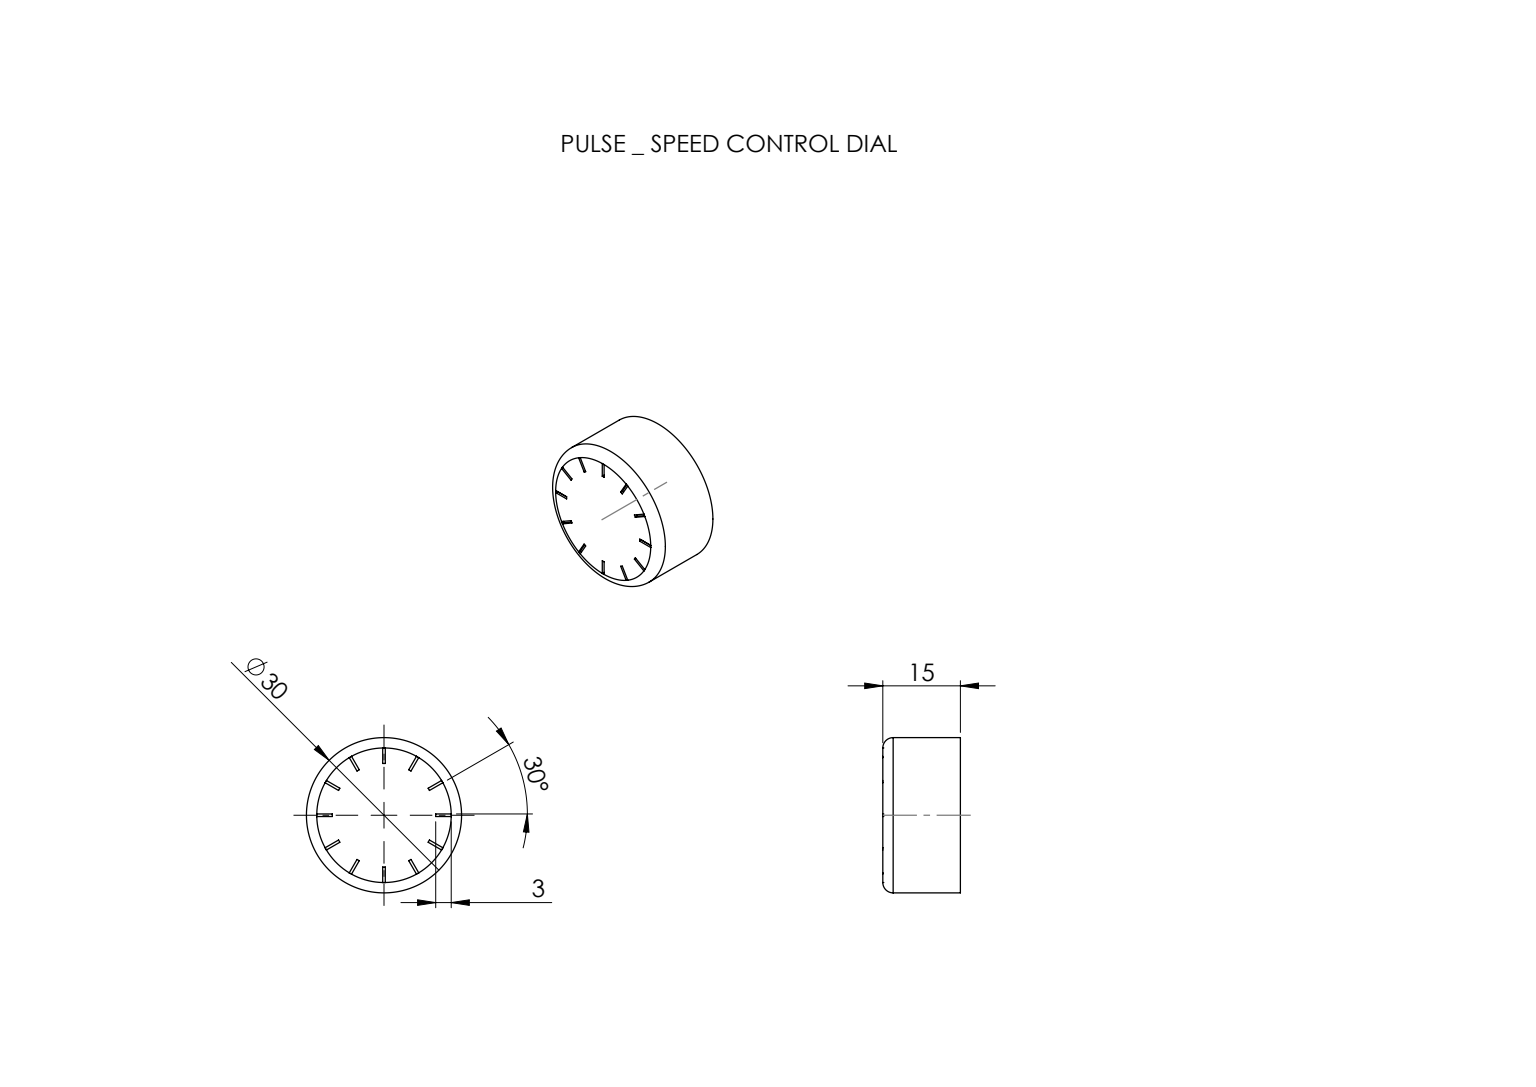
ISO-10303-21;
HEADER;
FILE_DESCRIPTION (('STEP AP214'),
    '1' );
FILE_NAME ('Pulse _ Speed Control Dial.step',
    '2026-10-08T14:59:03',
    ( '' ),
    ( '' ),
    'SwSTEP 2.0',
    'SolidWorks 2026',
    '' );
FILE_SCHEMA (( 'AUTOMOTIVE_DESIGN' ));
ENDSEC;

DATA;
#1=ORIENTED_EDGE ( 'NONE', *, *, #9406, .F. ) ;
#2=CARTESIAN_POINT ( 'NONE',  ( 11.80921887069467324, 30.25000000000018474, 79.50000000000000000 ) ) ;
#6=PLANE ( 'NONE',  #104 ) ;
#11=LINE ( 'NONE', #6448, #10967 ) ;
#15=ORIENTED_EDGE ( 'NONE', *, *, #10225, .T. ) ;
#17=ORIENTED_EDGE ( 'NONE', *, *, #3705, .T. ) ;
#19=EDGE_CURVE ( 'NONE', #6749, #65, #10302, .T. ) ;
#20=DIRECTION ( 'NONE',  ( 0.4999999999999933387, -0.8660254037844424824, 0.000000000000000000 ) ) ;
#21=ORIENTED_EDGE ( 'NONE', *, *, #5442, .F. ) ;
#22=VECTOR ( 'NONE', #10909, 1000.000000000000000 ) ;
#23=CARTESIAN_POINT ( 'NONE',  ( -7.907287480251413925, 18.86666975080236597, 80.00000000000000000 ) ) ;
#27=EDGE_CURVE ( 'NONE', #1251, #10198, #9485, .T. ) ;
#28=ORIENTED_EDGE ( 'NONE', *, *, #12033, .F. ) ;
#37=ORIENTED_EDGE ( 'NONE', *, *, #7691, .T. ) ;
#39=EDGE_CURVE ( 'NONE', #10896, #4898, #9360, .T. ) ;
#40=CARTESIAN_POINT ( 'NONE',  ( -1.440781129305471087, 43.00000000000008527, 80.00000000000000000 ) ) ;
#41=VECTOR ( 'NONE', #11324, 1000.000000000000000 ) ;
#45=VECTOR ( 'NONE', #2118, 1000.000000000000000 ) ;
#46=LINE ( 'NONE', #5798, #12120 ) ;
#47=LINE ( 'NONE', #9767, #6437 ) ;
#65=VERTEX_POINT ( 'NONE', #3417 ) ;
#67=ORIENTED_EDGE ( 'NONE', *, *, #12135, .T. ) ;
#73=CARTESIAN_POINT ( 'NONE',  ( 5.525725221640833240, 18.86666975080242992, 79.50000000000000000 ) ) ;
#78=AXIS2_PLACEMENT_3D ( 'NONE', #1523, #2574, #3573 ) ;
#82=CYLINDRICAL_SURFACE ( 'NONE', #2511, 15.00000000000000000 ) ;
#96=CARTESIAN_POINT ( 'NONE',  ( -1.440781129305282571, 17.00000000000009592, 80.00000000000000000 ) ) ;
#100=ORIENTED_EDGE ( 'NONE', *, *, #2094, .T. ) ;
#104=AXIS2_PLACEMENT_3D ( 'NONE', #11679, #5881, #9664 ) ;
#105=ORIENTED_EDGE ( 'NONE', *, *, #968, .F. ) ;
#110=DIRECTION ( 'NONE',  ( -0.8660254037844363761, 0.5000000000000038858, 0.000000000000000000 ) ) ;
#118=COLOUR_RGB ( '', 0.09019608, 0.27058824, 0.51372549) ;
#135=PLANE ( 'NONE',  #4004 ) ;
#139=ORIENTED_EDGE ( 'NONE', *, *, #323, .F. ) ;
#150=CARTESIAN_POINT ( 'NONE',  ( -0.9407811293052614765, 20.00000000000009237, 79.50000000000000000 ) ) ;
#156=ORIENTED_EDGE ( 'NONE', *, *, #11948, .T. ) ;
#159=CARTESIAN_POINT ( 'NONE',  ( 9.942549119892305498, 36.71650635094628967, 79.50000000000000000 ) ) ;
#160=MECHANICAL_DESIGN_GEOMETRIC_PRESENTATION_REPRESENTATION('',(#10913),#2162);
#162=ORIENTED_EDGE ( 'NONE', *, *, #3844, .F. ) ;
#168=ORIENTED_EDGE ( 'NONE', *, *, #9268, .F. ) ;
#169=CARTESIAN_POINT ( 'NONE',  ( -9.976035167149731819, 34.78349364905394481, 80.00000000000000000 ) ) ;
#171=LINE ( 'NONE', #7782, #5342 ) ;
#175=EDGE_CURVE ( 'NONE', #10718, #2926, #1576, .T. ) ;
#180=CARTESIAN_POINT ( 'NONE',  ( 11.80921887069467324, 30.00000000000008882, 80.00000000000000000 ) ) ;
#186=ORIENTED_EDGE ( 'NONE', *, *, #175, .F. ) ;
#187=DIRECTION ( 'NONE',  ( -1.000000000000000000, 0.000000000000000000, -0.000000000000000000 ) ) ;
#191=DIRECTION ( 'NONE',  ( -0.5000000000000095479, -0.8660254037844331565, 0.000000000000000000 ) ) ;
#195=DIRECTION ( 'NONE',  ( -0.000000000000000000, -0.000000000000000000, 1.000000000000000000 ) ) ;
#197=VECTOR ( 'NONE', #4605, 1000.000000000000000 ) ;
#200=EDGE_CURVE ( 'NONE', #12119, #9588, #3746, .T. ) ;
#204=VECTOR ( 'NONE', #4922, 1000.000000000000227 ) ;
#213=CARTESIAN_POINT ( 'NONE',  ( -7.473072744137204459, 18.61875173514729198, 80.00000000000000000 ) ) ;
#214=EDGE_CURVE ( 'NONE', #4965, #8588, #3628, .T. ) ;
#215=EDGE_CURVE ( 'NONE', #8652, #10794, #4622, .T. ) ;
#220=ORIENTED_EDGE ( 'NONE', *, *, #6316, .F. ) ;
#237=LINE ( 'NONE', #3111, #10805 ) ;
#240=CARTESIAN_POINT ( 'NONE',  ( -12.32411137850303184, 36.71650635094619730, 80.00000000000000000 ) ) ;
#242=AXIS2_PLACEMENT_3D ( 'NONE', #11636, #6579, #4023 ) ;
#243=CARTESIAN_POINT ( 'NONE',  ( -7.474274778359198734, 41.38333024919781167, 79.50000000000000000 ) ) ;
#255=ORIENTED_EDGE ( 'NONE', *, *, #4089, .F. ) ;
#264=CARTESIAN_POINT ( 'NONE',  ( -7.474274778359198734, 41.38333024919781167, 80.00000000000000000 ) ) ;
#271=FACE_OUTER_BOUND ( 'NONE', #1182, .T. ) ;
#275=CARTESIAN_POINT ( 'NONE',  ( -12.57411137850303540, 36.28349364905398033, 80.00000000000000000 ) ) ;
#277=EDGE_CURVE ( 'NONE', #893, #11323, #5445, .T. ) ;
#284=DIRECTION ( 'NONE',  ( -1.000000000000000000, 0.000000000000000000, 0.000000000000000000 ) ) ;
#295=ADVANCED_FACE ( 'NONE', ( #10535 ), #3875, .F. ) ;
#296=ORIENTED_EDGE ( 'NONE', *, *, #2512, .T. ) ;
#297=CARTESIAN_POINT ( 'NONE',  ( -7.474274778359196070, 18.61666975080236597, 79.50000000000000000 ) ) ;
#301=VERTEX_POINT ( 'NONE', #9472 ) ;
#313=CARTESIAN_POINT ( 'NONE',  ( 8.809218870694669690, 30.25000000000019540, 79.50000000000000000 ) ) ;
#315=ORIENTED_EDGE ( 'NONE', *, *, #5726, .F. ) ;
#316=CARTESIAN_POINT ( 'NONE',  ( 9.940467135547327970, 23.28469568327612649, 80.00000000000000000 ) ) ;
#323=EDGE_CURVE ( 'NONE', #2842, #3092, #6377, .T. ) ;
#332=LINE ( 'NONE', #5020, #6258 ) ;
#336=CARTESIAN_POINT ( 'NONE',  ( 11.80921887069467324, 30.25000000000018474, 79.50000000000000000 ) ) ;
#344=DIRECTION ( 'NONE',  ( 0.000000000000000000, 0.000000000000000000, 1.000000000000000000 ) ) ;
#349=DIRECTION ( 'NONE',  ( 0.8660254037844399289, 0.4999999999999977796, 0.000000000000000000 ) ) ;
#352=ORIENTED_EDGE ( 'NONE', *, *, #1928, .T. ) ;
#355=VECTOR ( 'NONE', #3125, 1000.000000000000000 ) ;
#358=LINE ( 'NONE', #7956, #6249 ) ;
#369=ORIENTED_EDGE ( 'NONE', *, *, #7765, .T. ) ;
#371=DIRECTION ( 'NONE',  ( 1.000000000000000000, 0.000000000000000000, 0.000000000000000000 ) ) ;
#372=ORIENTED_EDGE ( 'NONE', *, *, #5442, .T. ) ;
#377=ADVANCED_FACE ( 'NONE', ( #6817 ), #11436, .F. ) ;
#378=DIRECTION ( 'NONE',  ( 0.000000000000000000, 0.000000000000000000, -1.000000000000000000 ) ) ;
#379=DIRECTION ( 'NONE',  ( -0.8660254037844363761, 0.5000000000000038858, 0.000000000000000000 ) ) ;
#389=CARTESIAN_POINT ( 'NONE',  ( 0.000000000000000000, 0.000000000000000000, 79.50000000000000000 ) ) ;
#392=CARTESIAN_POINT ( 'NONE',  ( 7.594472908539098732, 25.21650635094628257, 79.50000000000000000 ) ) ;
#394=ORIENTED_EDGE ( 'NONE', *, *, #6090, .T. ) ;
#399=CARTESIAN_POINT ( 'NONE',  ( -14.19078112930533209, 29.75000000000008882, 80.00000000000000000 ) ) ;
#401=ORIENTED_EDGE ( 'NONE', *, *, #8827, .T. ) ;
#407=CARTESIAN_POINT ( 'NONE',  ( 7.344472908538985045, 35.21650635094629678, 80.00000000000000000 ) ) ;
#410=AXIS2_PLACEMENT_3D ( 'NONE', #11253, #12309, #8485 ) ;
#423=ORIENTED_EDGE ( 'NONE', *, *, #513, .F. ) ;
#428=CARTESIAN_POINT ( 'NONE',  ( -5.974274778359230709, 38.78525403784446723, 79.50000000000000000 ) ) ;
#434=VERTEX_POINT ( 'NONE', #4950 ) ;
#449=EDGE_CURVE ( 'NONE', #11346, #9412, #9727, .T. ) ;
#452=LINE ( 'NONE', #8050, #6872 ) ;
#457=ORIENTED_EDGE ( 'NONE', *, *, #2614, .F. ) ;
#464=ORIENTED_EDGE ( 'NONE', *, *, #4771, .T. ) ;
#467=DIRECTION ( 'NONE',  ( -0.8660254037844398178, -0.4999999999999977796, 0.000000000000000000 ) ) ;
#468=LINE ( 'NONE', #7942, #9415 ) ;
#469=LINE ( 'NONE', #10759, #4021 ) ;
#470=DIRECTION ( 'NONE',  ( -0.000000000000000000, -0.000000000000000000, -1.000000000000000000 ) ) ;
#476=ADVANCED_FACE ( 'NONE', ( #7582 ), #2973, .T. ) ;
#486=LINE ( 'NONE', #3166, #7436 ) ;
#488=DIRECTION ( 'NONE',  ( 0.000000000000000000, 0.000000000000000000, -1.000000000000000000 ) ) ;
#496=AXIS2_PLACEMENT_3D ( 'NONE', #3452, #10924, #1457 ) ;
#508=ORIENTED_EDGE ( 'NONE', *, *, #996, .T. ) ;
#510=EDGE_CURVE ( 'NONE', #4808, #2880, #3913, .T. ) ;
#513=EDGE_CURVE ( 'NONE', #872, #9323, #1788, .T. ) ;
#517=CARTESIAN_POINT ( 'NONE',  ( -5.974274778359230709, 38.78525403784446723, 80.00000000000000000 ) ) ;
#518=ORIENTED_EDGE ( 'NONE', *, *, #9580, .T. ) ;
#531=VECTOR ( 'NONE', #4205, 1000.000000000000000 ) ;
#533=CARTESIAN_POINT ( 'NONE',  ( 7.594472908538985045, 34.78349364905407270, 79.50000000000000000 ) ) ;
#539=CARTESIAN_POINT ( 'NONE',  ( -11.19078112930532498, 30.25000000000005684, 80.00000000000000000 ) ) ;
#542=LINE ( 'NONE', #4340, #4784 ) ;
#546=LINE ( 'NONE', #9891, #5841 ) ;
#563=ORIENTED_EDGE ( 'NONE', *, *, #4830, .F. ) ;
#574=EDGE_LOOP ( 'NONE', ( #9840, #12059, #508, #10243, #1092 ) ) ;
#578=EDGE_LOOP ( 'NONE', ( #7010, #3876, #2369, #10990, #1797 ) ) ;
#588=AXIS2_PLACEMENT_3D ( 'NONE', #8725, #5694, #11492 ) ;
#590=VERTEX_POINT ( 'NONE', #1349 ) ;
#596=EDGE_CURVE ( 'NONE', #11323, #590, #4560, .T. ) ;
#608=EDGE_CURVE ( 'NONE', #8652, #9323, #6330, .T. ) ;
#610=CARTESIAN_POINT ( 'NONE',  ( -1.107447795970746940, 43.00000000000008527, 80.00000000000000000 ) ) ;
#611=ORIENTED_EDGE ( 'NONE', *, *, #12343, .T. ) ;
#616=PLANE ( 'NONE',  #7657 ) ;
#619=CARTESIAN_POINT ( 'NONE',  ( -9.976035167149731819, 34.78349364905394481, 79.50000000000000000 ) ) ;
#624=ORIENTED_EDGE ( 'NONE', *, *, #6789, .F. ) ;
#632=VERTEX_POINT ( 'NONE', #11072 ) ;
#636=ORIENTED_EDGE ( 'NONE', *, *, #12117, .T. ) ;
#643=EDGE_CURVE ( 'NONE', #2035, #9573, #11004, .T. ) ;
#650=ORIENTED_EDGE ( 'NONE', *, *, #2819, .T. ) ;
#667=EDGE_LOOP ( 'NONE', ( #12006, #10960, #1141, #1963 ) ) ;
#669=VECTOR ( 'NONE', #12025, 1000.000000000000000 ) ;
#678=EDGE_LOOP ( 'NONE', ( #186, #9403, #7670, #10826, #1970 ) ) ;
#680=LINE ( 'NONE', #8276, #8746 ) ;
#681=EDGE_CURVE ( 'NONE', #7265, #8236, #4523, .T. ) ;
#687=ORIENTED_EDGE ( 'NONE', *, *, #7241, .F. ) ;
#692=PLANE ( 'NONE',  #2879 ) ;
#698=PLANE ( 'NONE',  #5126 ) ;
#701=EDGE_CURVE ( 'NONE', #2446, #6472, #11195, .T. ) ;
#713=EDGE_CURVE ( 'NONE', #590, #6198, #8187, .T. ) ;
#716=EDGE_LOOP ( 'NONE', ( #6121, #4199, #2055, #8173 ) ) ;
#717=ADVANCED_FACE ( 'NONE', ( #8066 ), #12010, .T. ) ;
#739=PLANE ( 'NONE',  #9145 ) ;
#741=CARTESIAN_POINT ( 'NONE',  ( -1.190781129305471087, 43.00000000000008527, 80.00000000000000000 ) ) ;
#750=DIRECTION ( 'NONE',  ( -0.000000000000000000, -0.000000000000000000, 1.000000000000000000 ) ) ;
#756=ORIENTED_EDGE ( 'NONE', *, *, #4698, .F. ) ;
#760=ORIENTED_EDGE ( 'NONE', *, *, #3268, .T. ) ;
#764=CARTESIAN_POINT ( 'NONE',  ( -1.440781129305471087, 43.00000000000008527, 80.00000000000000000 ) ) ;
#774=LINE ( 'NONE', #11179, #7774 ) ;
#777=DIRECTION ( 'NONE',  ( 0.000000000000000000, 0.000000000000000000, 1.000000000000000000 ) ) ;
#779=ORIENTED_EDGE ( 'NONE', *, *, #2337, .T. ) ;
#783=CARTESIAN_POINT ( 'NONE',  ( -0.9407811293054709756, 43.00000000000008527, 80.00000000000000000 ) ) ;
#806=EDGE_LOOP ( 'NONE', ( #3816, #1259, #9132, #4908 ) ) ;
#810=PLANE ( 'NONE',  #2982 ) ;
#815=ORIENTED_EDGE ( 'NONE', *, *, #3454, .T. ) ;
#821=ORIENTED_EDGE ( 'NONE', *, *, #12135, .F. ) ;
#828=VERTEX_POINT ( 'NONE', #2897 ) ;
#832=EDGE_CURVE ( 'NONE', #6075, #1902, #4700, .T. ) ;
#835=DIRECTION ( 'NONE',  ( -0.000000000000000000, -0.000000000000000000, 1.000000000000000000 ) ) ;
#840=DIRECTION ( 'NONE',  ( -0.000000000000000000, -0.000000000000000000, 1.000000000000000000 ) ) ;
#844=EDGE_CURVE ( 'NONE', #867, #7067, #11236, .T. ) ;
#848=CARTESIAN_POINT ( 'NONE',  ( -7.474274778359196070, 18.61666975080236597, 79.50000000000000000 ) ) ;
#855=DIRECTION ( 'NONE',  ( 0.5000000000000066613, 0.8660254037844347108, 0.000000000000000000 ) ) ;
#862=PLANE ( 'NONE',  #11013 ) ;
#865=EDGE_CURVE ( 'NONE', #1902, #8652, #11263, .T. ) ;
#867=VERTEX_POINT ( 'NONE', #7454 ) ;
#871=CARTESIAN_POINT ( 'NONE',  ( 8.809218870694669690, 30.25000000000019540, 80.00000000000000000 ) ) ;
#872=VERTEX_POINT ( 'NONE', #1775 ) ;
#873=CARTESIAN_POINT ( 'NONE',  ( -5.974274778359230709, 38.78525403784446723, 79.50000000000000000 ) ) ;
#879=DIRECTION ( 'NONE',  ( 0.4999999999999933387, -0.8660254037844424824, 0.000000000000000000 ) ) ;
#880=ORIENTED_EDGE ( 'NONE', *, *, #11127, .T. ) ;
#882=LINE ( 'NONE', #3739, #11237 ) ;
#883=LINE ( 'NONE', #4804, #7408 ) ;
#884=PLANE ( 'NONE',  #9162 ) ;
#885=VECTOR ( 'NONE', #3261, 1000.000000000000000 ) ;
#888=AXIS2_PLACEMENT_3D ( 'NONE', #5286, #4097, #5226 ) ;
#893=VERTEX_POINT ( 'NONE', #5893 ) ;
#899=FACE_OUTER_BOUND ( 'NONE', #3260, .T. ) ;
#900=DIRECTION ( 'NONE',  ( -0.000000000000000000, -0.000000000000000000, 1.000000000000000000 ) ) ;
#909=VECTOR ( 'NONE', #8508, 1000.000000000000114 ) ;
#914=VECTOR ( 'NONE', #4848, 1000.000000000000114 ) ;
#916=CARTESIAN_POINT ( 'NONE',  ( -7.474274778359196070, 18.61666975080236597, 79.50000000000000000 ) ) ;
#919=ORIENTED_EDGE ( 'NONE', *, *, #10882, .F. ) ;
#925=ORIENTED_EDGE ( 'NONE', *, *, #449, .T. ) ;
#927=EDGE_CURVE ( 'NONE', #9416, #10602, #9613, .T. ) ;
#935=DIRECTION ( 'NONE',  ( 0.000000000000000000, 0.000000000000000000, 1.000000000000000000 ) ) ;
#938=VERTEX_POINT ( 'NONE', #4137 ) ;
#953=EDGE_CURVE ( 'NONE', #9323, #9030, #7991, .T. ) ;
#967=( LENGTH_UNIT ( ) NAMED_UNIT ( * ) SI_UNIT ( .MILLI., .METRE. ) );
#968=EDGE_CURVE ( 'NONE', #9588, #4898, #3082, .T. ) ;
#969=VECTOR ( 'NONE', #11600, 1000.000000000000114 ) ;
#972=DIRECTION ( 'NONE',  ( 0.000000000000000000, 0.000000000000000000, 1.000000000000000000 ) ) ;
#975=ORIENTED_EDGE ( 'NONE', *, *, #7214, .F. ) ;
#984=EDGE_LOOP ( 'NONE', ( #5661, #255, #2855, #6607 ) ) ;
#985=LINE ( 'NONE', #159, #4247 ) ;
#996=EDGE_CURVE ( 'NONE', #10179, #5363, #332, .T. ) ;
#997=EDGE_CURVE ( 'NONE', #2035, #8327, #8801, .T. ) ;
#1000=AXIS2_PLACEMENT_3D ( 'NONE', #873, #12220, #7534 ) ;
#1012=ORIENTED_EDGE ( 'NONE', *, *, #175, .T. ) ;
#1024=CARTESIAN_POINT ( 'NONE',  ( -14.19078112930532853, 30.25000000000008882, 80.00000000000000000 ) ) ;
#1043=LINE ( 'NONE', #5844, #11222 ) ;
#1046=DIRECTION ( 'NONE',  ( 0.4999999999999933387, -0.8660254037844424824, 0.000000000000000000 ) ) ;
#1050=VECTOR ( 'NONE', #3209, 1000.000000000000000 ) ;
#1051=ADVANCED_FACE ( 'NONE', ( #8112 ), #8052, .T. ) ;
#1054=ORIENTED_EDGE ( 'NONE', *, *, #10513, .F. ) ;
#1060=ORIENTED_EDGE ( 'NONE', *, *, #9142, .F. ) ;
#1073=DIRECTION ( 'NONE',  ( -0.000000000000000000, 0.000000000000000000, 1.000000000000000000 ) ) ;
#1079=EDGE_CURVE ( 'NONE', #10836, #11969, #1581, .T. ) ;
#1092=ORIENTED_EDGE ( 'NONE', *, *, #2427, .F. ) ;
#1094=DIRECTION ( 'NONE',  ( -1.000000000000000000, 0.000000000000000000, 0.000000000000000000 ) ) ;
#1098=CARTESIAN_POINT ( 'NONE',  ( 9.942549119892305498, 36.71650635094628967, 79.50000000000000000 ) ) ;
#1101=ORIENTED_EDGE ( 'NONE', *, *, #7916, .T. ) ;
#1118=LINE ( 'NONE', #9764, #7955 ) ;
#1124=ORIENTED_EDGE ( 'NONE', *, *, #5258, .T. ) ;
#1135=VECTOR ( 'NONE', #379, 1000.000000000000114 ) ;
#1136=ORIENTED_EDGE ( 'NONE', *, *, #4089, .T. ) ;
#1141=ORIENTED_EDGE ( 'NONE', *, *, #11763, .T. ) ;
#1161=ORIENTED_EDGE ( 'NONE', *, *, #3154, .T. ) ;
#1170=CARTESIAN_POINT ( 'NONE',  ( -1.440781129305282571, 17.00000000000009592, 79.50000000000000000 ) ) ;
#1175=CARTESIAN_POINT ( 'NONE',  ( -7.907287480251421030, 41.13333024919781167, 80.00000000000000000 ) ) ;
#1176=EDGE_CURVE ( 'NONE', #7950, #1521, #6563, .T. ) ;
#1179=ORIENTED_EDGE ( 'NONE', *, *, #11127, .F. ) ;
#1182=EDGE_LOOP ( 'NONE', ( #9699, #464, #7429, #10894 ) ) ;
#1190=CIRCLE ( 'NONE', #1215, 12.99999999999999822 ) ;
#1197=DIRECTION ( 'NONE',  ( 0.4999999999999878431, -0.8660254037844455910, 0.000000000000000000 ) ) ;
#1199=VERTEX_POINT ( 'NONE', #3692 ) ;
#1204=DIRECTION ( 'NONE',  ( -0.8660254037844363761, 0.5000000000000038858, 0.000000000000000000 ) ) ;
#1205=DIRECTION ( 'NONE',  ( -0.000000000000000000, -1.000000000000000000, 0.000000000000000000 ) ) ;
#1207=CARTESIAN_POINT ( 'NONE',  ( -12.57411137850303540, 36.28349364905398033, 79.50000000000000000 ) ) ;
#1212=ORIENTED_EDGE ( 'NONE', *, *, #9053, .T. ) ;
#1215=AXIS2_PLACEMENT_3D ( 'NONE', #7760, #3839, #7636 ) ;
#1225=VECTOR ( 'NONE', #7313, 1000.000000000000227 ) ;
#1237=LINE ( 'NONE', #1924, #204 ) ;
#1251=VERTEX_POINT ( 'NONE', #6624 ) ;
#1259=ORIENTED_EDGE ( 'NONE', *, *, #11128, .F. ) ;
#1260=FACE_OUTER_BOUND ( 'NONE', #11178, .T. ) ;
#1262=ORIENTED_EDGE ( 'NONE', *, *, #11781, .T. ) ;
#1264=LINE ( 'NONE', #10854, #1135 ) ;
#1265=PLANE ( 'NONE',  #4606 ) ;
#1270=ORIENTED_EDGE ( 'NONE', *, *, #7421, .F. ) ;
#1288=EDGE_CURVE ( 'NONE', #6190, #9044, #12187, .T. ) ;
#1291=VECTOR ( 'NONE', #3516, 1000.000000000000114 ) ;
#1300=B_SPLINE_CURVE_WITH_KNOTS ( 'NONE', 3,
 ( #180, #7730, #11608, #4735 ),
 .UNSPECIFIED., .F., .F.,
 ( 4, 4 ),
 ( 0.0009573067811866411980, 0.001207306781186544276 ),
 .UNSPECIFIED. ) ;
#1305=ORIENTED_EDGE ( 'NONE', *, *, #4806, .T. ) ;
#1312=VERTEX_POINT ( 'NONE', #316 ) ;
#1320=ORIENTED_EDGE ( 'NONE', *, *, #2719, .F. ) ;
#1322=DIRECTION ( 'NONE',  ( 0.8660254037844394848, -0.4999999999999985567, 0.000000000000000000 ) ) ;
#1334=ORIENTED_EDGE ( 'NONE', *, *, #9809, .T. ) ;
#1341=LINE ( 'NONE', #8869, #1050 ) ;
#1348=EDGE_LOOP ( 'NONE', ( #9516, #8341, #6017, #6615, #423 ) ) ;
#1349=CARTESIAN_POINT ( 'NONE',  ( 10.19254911989230727, 36.28349364905406560, 80.00000000000000000 ) ) ;
#1351=DIRECTION ( 'NONE',  ( 0.000000000000000000, 0.000000000000000000, -1.000000000000000000 ) ) ;
#1361=ORIENTED_EDGE ( 'NONE', *, *, #4938, .F. ) ;
#1362=DIRECTION ( 'NONE',  ( -0.000000000000000000, -0.000000000000000000, 1.000000000000000000 ) ) ;
#1370=EDGE_CURVE ( 'NONE', #11096, #11491, #11678, .T. ) ;
#1372=VERTEX_POINT ( 'NONE', #4943 ) ;
#1385=ORIENTED_EDGE ( 'NONE', *, *, #643, .T. ) ;
#1389=VECTOR ( 'NONE', #6685, 1000.000000000000000 ) ;
#1401=LINE ( 'NONE', #336, #3404 ) ;
#1403=CARTESIAN_POINT ( 'NONE',  ( -12.32411137850302119, 23.28349364905396612, 79.50000000000000000 ) ) ;
#1416=VECTOR ( 'NONE', #6438, 1000.000000000000000 ) ;
#1420=VERTEX_POINT ( 'NONE', #10544 ) ;
#1421=CARTESIAN_POINT ( 'NONE',  ( -7.907287480251421030, 41.13333024919781167, 80.00000000000000000 ) ) ;
#1431=EDGE_CURVE ( 'NONE', #1372, #1941, #9785, .T. ) ;
#1432=LINE ( 'NONE', #10900, #5872 ) ;
#1433=ADVANCED_FACE ( 'NONE', ( #1260 ), #5070, .T. ) ;
#1444=CARTESIAN_POINT ( 'NONE',  ( 3.592712519748450628, 38.78525403784453118, 79.50000000000000000 ) ) ;
#1457=DIRECTION ( 'NONE',  ( 1.000000000000000000, -1.387778780781445676E-14, 0.000000000000000000 ) ) ;
#1465=DIRECTION ( 'NONE',  ( -0.000000000000000000, -0.000000000000000000, 1.000000000000000000 ) ) ;
#1468=VERTEX_POINT ( 'NONE', #5433 ) ;
#1470=ORIENTED_EDGE ( 'NONE', *, *, #2038, .T. ) ;
#1471=AXIS2_PLACEMENT_3D ( 'NONE', #2725, #1790, #9382 ) ;
#1487=ORIENTED_EDGE ( 'NONE', *, *, #4666, .F. ) ;
#1504=VECTOR ( 'NONE', #2164, 1000.000000000000000 ) ;
#1505=ORIENTED_EDGE ( 'NONE', *, *, #10254, .F. ) ;
#1506=CARTESIAN_POINT ( 'NONE',  ( 3.592712519748450628, 38.78525403784453118, 80.00000000000000000 ) ) ;
#1509=DIRECTION ( 'NONE',  ( -1.000000000000000000, 0.000000000000000000, -0.000000000000000000 ) ) ;
#1511=CARTESIAN_POINT ( 'NONE',  ( -6.407287480251453893, 38.53525403784446723, 79.50000000000000000 ) ) ;
#1521=VERTEX_POINT ( 'NONE', #1506 ) ;
#1522=B_SPLINE_CURVE_WITH_KNOTS ( 'NONE', 3,
 ( #9804, #4141, #7131, #6078 ),
 .UNSPECIFIED., .F., .F.,
 ( 4, 4 ),
 ( 0.0002502309401078863893, 0.0005002309401076776314 ),
 .UNSPECIFIED. ) ;
#1523=CARTESIAN_POINT ( 'NONE',  ( 5.092712519748611832, 18.61666975080242992, 79.50000000000000000 ) ) ;
#1533=ORIENTED_EDGE ( 'NONE', *, *, #1370, .T. ) ;
#1536=DIRECTION ( 'NONE',  ( -0.000000000000000000, -0.000000000000000000, -1.000000000000000000 ) ) ;
#1539=DIRECTION ( 'NONE',  ( 7.011174048739587977E-15, 1.000000000000000000, 0.000000000000000000 ) ) ;
#1540=CARTESIAN_POINT ( 'NONE',  ( -14.19078112930532853, 30.25000000000008882, 80.00000000000000000 ) ) ;
#1549=CARTESIAN_POINT ( 'NONE',  ( 5.092712519748452848, 41.38333024919784719, 79.50000000000000000 ) ) ;
#1551=EDGE_CURVE ( 'NONE', #5535, #9044, #6178, .T. ) ;
#1552=CARTESIAN_POINT ( 'NONE',  ( -7.907287480251413925, 18.86666975080236597, 80.00000000000000000 ) ) ;
#1553=ADVANCED_FACE ( 'NONE', ( #4241 ), #8097, .F. ) ;
#1566=DIRECTION ( 'NONE',  ( -0.4999999999999942268, 0.8660254037844419273, 0.000000000000000000 ) ) ;
#1571=CARTESIAN_POINT ( 'NONE',  ( 0.000000000000000000, 0.000000000000000000, 79.50000000000000000 ) ) ;
#1574=VERTEX_POINT ( 'NONE', #2437 ) ;
#1576=LINE ( 'NONE', #1759, #3413 ) ;
#1581=LINE ( 'NONE', #7381, #11442 ) ;
#1586=CARTESIAN_POINT ( 'NONE',  ( 5.525725221640833240, 18.86666975080242992, 79.50000000000000000 ) ) ;
#1598=EDGE_CURVE ( 'NONE', #9749, #8477, #6304, .T. ) ;
#1605=VECTOR ( 'NONE', #3418, 1000.000000000000114 ) ;
#1606=DIRECTION ( 'NONE',  ( -0.8660254037844363761, 0.5000000000000038858, 0.000000000000000000 ) ) ;
#1609=ORIENTED_EDGE ( 'NONE', *, *, #3387, .F. ) ;
#1611=EDGE_CURVE ( 'NONE', #1631, #10896, #4549, .T. ) ;
#1612=AXIS2_PLACEMENT_3D ( 'NONE', #9562, #7823, #5032 ) ;
#1621=VECTOR ( 'NONE', #9526, 1000.000000000000000 ) ;
#1625=ORIENTED_EDGE ( 'NONE', *, *, #7141, .T. ) ;
#1631=VERTEX_POINT ( 'NONE', #4491 ) ;
#1635=CARTESIAN_POINT ( 'NONE',  ( -0.9407811293052825707, 17.00000000000008882, 79.50000000000000000 ) ) ;
#1639=ADVANCED_FACE ( 'NONE', ( #3915 ), #10515, .T. ) ;
#1654=CIRCLE ( 'NONE', #10398, 14.99999999999999822 ) ;
#1655=EDGE_CURVE ( 'NONE', #8730, #5158, #12108, .T. ) ;
#1660=DIRECTION ( 'NONE',  ( -0.000000000000000000, -0.000000000000000000, 1.000000000000000000 ) ) ;
#1678=DIRECTION ( 'NONE',  ( 1.000000000000000000, 0.000000000000000000, 0.000000000000000000 ) ) ;
#1680=FACE_OUTER_BOUND ( 'NONE', #11150, .T. ) ;
#1691=ORIENTED_EDGE ( 'NONE', *, *, #12343, .F. ) ;
#1696=AXIS2_PLACEMENT_3D ( 'NONE', #11366, #10355, #4686 ) ;
#1699=ORIENTED_EDGE ( 'NONE', *, *, #1288, .T. ) ;
#1721=CARTESIAN_POINT ( 'NONE',  ( 10.19254911989230727, 36.28349364905406560, 80.00000000000000000 ) ) ;
#1726=CARTESIAN_POINT ( 'NONE',  ( -1.190781129305651387, 17.00000000000009237, 80.00000000000000000 ) ) ;
#1759=CARTESIAN_POINT ( 'NONE',  ( -7.474274778359196070, 18.61666975080236597, 80.00000000000000000 ) ) ;
#1762=DIRECTION ( 'NONE',  ( -1.000000000000000000, 3.469446951953611033E-15, 0.000000000000000000 ) ) ;
#1767=ORIENTED_EDGE ( 'NONE', *, *, #8553, .F. ) ;
#1775=CARTESIAN_POINT ( 'NONE',  ( -7.906085446029426755, 18.86875173514728488, 80.00000000000000000 ) ) ;
#1779=EDGE_CURVE ( 'NONE', #301, #3643, #469, .T. ) ;
#1786=CIRCLE ( 'NONE', #8147, 12.99999999999999822 ) ;
#1788=LINE ( 'NONE', #2723, #909 ) ;
#1790=DIRECTION ( 'NONE',  ( 0.000000000000000000, 0.000000000000000000, 1.000000000000000000 ) ) ;
#1796=CARTESIAN_POINT ( 'NONE',  ( -0.9407811293052825707, 17.00000000000008882, 80.00000000000000000 ) ) ;
#1797=ORIENTED_EDGE ( 'NONE', *, *, #1926, .F. ) ;
#1810=EDGE_LOOP ( 'NONE', ( #105, #3051, #1136, #6544 ) ) ;
#1823=CARTESIAN_POINT ( 'NONE',  ( -1.190781129305651387, 17.00000000000009237, 80.00000000000000000 ) ) ;
#1829=LINE ( 'NONE', #5639, #7508 ) ;
#1830=FACE_OUTER_BOUND ( 'NONE', #7383, .T. ) ;
#1833=DIRECTION ( 'NONE',  ( -0.000000000000000000, -0.000000000000000000, 1.000000000000000000 ) ) ;
#1835=ADVANCED_FACE ( 'NONE', ( #2283 ), #9754, .F. ) ;
#1842=FACE_OUTER_BOUND ( 'NONE', #10044, .T. ) ;
#1863=CARTESIAN_POINT ( 'NONE',  ( 9.942549119892413856, 23.28349364905404428, 80.00000000000000000 ) ) ;
#1867=ORIENTED_EDGE ( 'NONE', *, *, #7605, .F. ) ;
#1871=ADVANCED_FACE ( 'NONE', ( #5222 ), #8005, .T. ) ;
#1887=LINE ( 'NONE', #3013, #5916 ) ;
#1902=VERTEX_POINT ( 'NONE', #7086 ) ;
#1907=EDGE_CURVE ( 'NONE', #301, #5980, #6149, .T. ) ;
#1916=ORIENTED_EDGE ( 'NONE', *, *, #9580, .F. ) ;
#1917=LINE ( 'NONE', #7586, #3656 ) ;
#1920=FACE_OUTER_BOUND ( 'NONE', #7935, .T. ) ;
#1922=LINE ( 'NONE', #4919, #4271 ) ;
#1923=ORIENTED_EDGE ( 'NONE', *, *, #4088, .F. ) ;
#1924=CARTESIAN_POINT ( 'NONE',  ( 4.025725221640669815, 38.53525403784453118, 80.00000000000000000 ) ) ;
#1926=EDGE_CURVE ( 'NONE', #8236, #8588, #7273, .T. ) ;
#1928=EDGE_CURVE ( 'NONE', #10032, #9030, #3589, .T. ) ;
#1929=CARTESIAN_POINT ( 'NONE',  ( -12.57411137850303540, 36.28349364905398033, 79.50000000000000000 ) ) ;
#1931=ORIENTED_EDGE ( 'NONE', *, *, #2094, .F. ) ;
#1941=VERTEX_POINT ( 'NONE', #11134 ) ;
#1960=VERTEX_POINT ( 'NONE', #11199 ) ;
#1963=ORIENTED_EDGE ( 'NONE', *, *, #701, .F. ) ;
#1965=DIRECTION ( 'NONE',  ( -0.4999999999999985012, -0.8660254037844394848, 0.000000000000000000 ) ) ;
#1968=CARTESIAN_POINT ( 'NONE',  ( 9.942549119892305498, 36.71650635094628967, 79.50000000000000000 ) ) ;
#1970=ORIENTED_EDGE ( 'NONE', *, *, #4392, .F. ) ;
#1972=EDGE_CURVE ( 'NONE', #8477, #5671, #3650, .T. ) ;
#1975=CARTESIAN_POINT ( 'NONE',  ( 5.092712519748611832, 18.61666975080242992, 79.50000000000000000 ) ) ;
#1979=ORIENTED_EDGE ( 'NONE', *, *, #215, .F. ) ;
#1980=PLANE ( 'NONE',  #888 ) ;
#1981=DIRECTION ( 'NONE',  ( 0.000000000000000000, 0.000000000000000000, 1.000000000000000000 ) ) ;
#1983=VECTOR ( 'NONE', #835, 1000.000000000000000 ) ;
#1984=ORIENTED_EDGE ( 'NONE', *, *, #9038, .T. ) ;
#1990=DIRECTION ( 'NONE',  ( -0.4999999999999942268, 0.8660254037844419273, 0.000000000000000000 ) ) ;
#1994=PLANE ( 'NONE',  #4105 ) ;
#2000=ORIENTED_EDGE ( 'NONE', *, *, #11440, .T. ) ;
#2016=LINE ( 'NONE', #7864, #10761 ) ;
#2017=DIRECTION ( 'NONE',  ( 0.8660254037844420383, 0.4999999999999942824, 0.000000000000000000 ) ) ;
#2022=ORIENTED_EDGE ( 'NONE', *, *, #8900, .F. ) ;
#2023=PRESENTATION_STYLE_ASSIGNMENT (( #10618 ) ) ;
#2035=VERTEX_POINT ( 'NONE', #6214 ) ;
#2038=EDGE_CURVE ( 'NONE', #2522, #434, #7207, .T. ) ;
#2045=DIRECTION ( 'NONE',  ( -0.4999999999999942268, 0.8660254037844419273, 0.000000000000000000 ) ) ;
#2046=CARTESIAN_POINT ( 'NONE',  ( -11.19078112930532498, 30.25000000000005684, 79.50000000000000000 ) ) ;
#2048=EDGE_LOOP ( 'NONE', ( #7070, #1054, #7481, #6311 ) ) ;
#2053=DIRECTION ( 'NONE',  ( -0.8660254037844394848, -0.4999999999999985567, 0.000000000000000000 ) ) ;
#2055=ORIENTED_EDGE ( 'NONE', *, *, #2920, .F. ) ;
#2067=ORIENTED_EDGE ( 'NONE', *, *, #3141, .F. ) ;
#2068=PLANE ( 'NONE',  #8935 ) ;
#2072=FACE_OUTER_BOUND ( 'NONE', #6725, .T. ) ;
#2073=ORIENTED_EDGE ( 'NONE', *, *, #8808, .F. ) ;
#2077=DIRECTION ( 'NONE',  ( -0.5000000000000006661, -0.8660254037844383745, 0.000000000000000000 ) ) ;
#2080=CARTESIAN_POINT ( 'NONE',  ( -7.546443561989872428, 41.34166358254155682, 80.00000048127353125 ) ) ;
#2082=( NAMED_UNIT ( * ) PLANE_ANGLE_UNIT ( ) SI_UNIT ( $, .RADIAN. ) );
#2084=VERTEX_POINT ( 'NONE', #4705 ) ;
#2094=EDGE_CURVE ( 'NONE', #7950, #6913, #1190, .T. ) ;
#2106=CARTESIAN_POINT ( 'NONE',  ( -12.32411137850302119, 23.28349364905396612, 80.00000000000000000 ) ) ;
#2111=CARTESIAN_POINT ( 'NONE',  ( 11.80921887069452580, 30.00000000000008882, 78.00000000000000000 ) ) ;
#2118=DIRECTION ( 'NONE',  ( -0.000000000000000000, -0.000000000000000000, 1.000000000000000000 ) ) ;
#2120=CARTESIAN_POINT ( 'NONE',  ( -1.190781129305471087, 30.00000000000008882, 80.00000000000000000 ) ) ;
#2124=CARTESIAN_POINT ( 'NONE',  ( -9.726035167149728267, 35.21650635094616888, 80.00000000000000000 ) ) ;
#2126=ORIENTED_EDGE ( 'NONE', *, *, #277, .T. ) ;
#2132=CARTESIAN_POINT ( 'NONE',  ( 9.942549119892305498, 36.71650635094628967, 80.00000000000000000 ) ) ;
#2140=LINE ( 'NONE', #1024, #5199 ) ;
#2145=ORIENTED_EDGE ( 'NONE', *, *, #510, .T. ) ;
#2151=CARTESIAN_POINT ( 'NONE',  ( -12.44911137850304250, 36.50000000000007816, 80.00000000000000000 ) ) ;
#2162=( GEOMETRIC_REPRESENTATION_CONTEXT ( 3 ) GLOBAL_UNCERTAINTY_ASSIGNED_CONTEXT ( ( #7522 ) ) GLOBAL_UNIT_ASSIGNED_CONTEXT ( ( #5830, #2082, #3956 ) ) REPRESENTATION_CONTEXT ( 'NONE', 'WORKASPACE' ) );
#2164=DIRECTION ( 'NONE',  ( -0.000000000000000000, -0.000000000000000000, 1.000000000000000000 ) ) ;
#2167=DIRECTION ( 'NONE',  ( 1.000000000000000000, 0.000000000000000000, 0.000000000000000000 ) ) ;
#2172=EDGE_LOOP ( 'NONE', ( #1385, #4057, #975, #1609, #12259 ) ) ;
#2174=CIRCLE ( 'NONE', #9126, 12.99999999999999822 ) ;
#2187=CARTESIAN_POINT ( 'NONE',  ( -16.19078112930547064, 30.00000000000008882, 65.00000000000000000 ) ) ;
#2193=LINE ( 'NONE', #3012, #9052 ) ;
#2195=FACE_OUTER_BOUND ( 'NONE', #5983, .T. ) ;
#2196=ORIENTED_EDGE ( 'NONE', *, *, #2512, .F. ) ;
#2199=EDGE_CURVE ( 'NONE', #6075, #10794, #11387, .T. ) ;
#2204=EDGE_LOOP ( 'NONE', ( #3819, #880, #11119, #3936, #1212 ) ) ;
#2216=ORIENTED_EDGE ( 'NONE', *, *, #6232, .F. ) ;
#2225=CARTESIAN_POINT ( 'NONE',  ( 9.942549119892413856, 23.28349364905404428, 80.00000000000000000 ) ) ;
#2226=CARTESIAN_POINT ( 'NONE',  ( -9.976035167149682081, 25.21650635094616533, 79.50000000000000000 ) ) ;
#2250=ORIENTED_EDGE ( 'NONE', *, *, #4793, .T. ) ;
#2252=CARTESIAN_POINT ( 'NONE',  ( -6.407287480251391720, 21.46474596215567487, 80.00000000000000000 ) ) ;
#2254=VECTOR ( 'NONE', #7647, 1000.000000000000000 ) ;
#2273=EDGE_CURVE ( 'NONE', #7990, #2035, #1401, .T. ) ;
#2274=VERTEX_POINT ( 'NONE', #6139 ) ;
#2282=AXIS2_PLACEMENT_3D ( 'NONE', #2664, #6475, #5356 ) ;
#2283=FACE_OUTER_BOUND ( 'NONE', #10867, .T. ) ;
#2295=FACE_OUTER_BOUND ( 'NONE', #3987, .T. ) ;
#2296=ORIENTED_EDGE ( 'NONE', *, *, #7572, .T. ) ;
#2302=ORIENTED_EDGE ( 'NONE', *, *, #7763, .F. ) ;
#2311=VERTEX_POINT ( 'NONE', #5898 ) ;
#2318=CARTESIAN_POINT ( 'NONE',  ( 5.309218870694559556, 41.25833024919784719, 80.00000000000000000 ) ) ;
#2325=CARTESIAN_POINT ( 'NONE',  ( -12.32411137850302119, 23.28349364905396612, 80.00000000000000000 ) ) ;
#2329=VERTEX_POINT ( 'NONE', #11758 ) ;
#2331=LINE ( 'NONE', #7821, #9326 ) ;
#2336=ORIENTED_EDGE ( 'NONE', *, *, #7763, .T. ) ;
#2337=EDGE_CURVE ( 'NONE', #1631, #9640, #2331, .T. ) ;
#2343=LINE ( 'NONE', #9063, #3912 ) ;
#2352=ORIENTED_EDGE ( 'NONE', *, *, #6920, .F. ) ;
#2357=ORIENTED_EDGE ( 'NONE', *, *, #9659, .F. ) ;
#2359=CARTESIAN_POINT ( 'NONE',  ( -1.440781129305471087, 40.00000000000008527, 79.50000000000000000 ) ) ;
#2360=ORIENTED_EDGE ( 'NONE', *, *, #7154, .T. ) ;
#2369=ORIENTED_EDGE ( 'NONE', *, *, #2920, .T. ) ;
#2370=CARTESIAN_POINT ( 'NONE',  ( -7.907287480251421030, 41.13333024919781167, 80.00000000000000000 ) ) ;
#2372=ORIENTED_EDGE ( 'NONE', *, *, #5795, .T. ) ;
#2375=FACE_OUTER_BOUND ( 'NONE', #2172, .T. ) ;
#2383=ORIENTED_EDGE ( 'NONE', *, *, #7916, .F. ) ;
#2393=ORIENTED_EDGE ( 'NONE', *, *, #6090, .F. ) ;
#2402=CARTESIAN_POINT ( 'NONE',  ( -12.57411137850303540, 36.28349364905398033, 80.00000000000000000 ) ) ;
#2403=VECTOR ( 'NONE', #7745, 1000.000000000000000 ) ;
#2419=FACE_OUTER_BOUND ( 'NONE', #4288, .T. ) ;
#2420=CARTESIAN_POINT ( 'NONE',  ( 5.453556438010031648, 41.17499691585408783, 80.00000048127353125 ) ) ;
#2427=EDGE_CURVE ( 'NONE', #3092, #11844, #774, .T. ) ;
#2435=ORIENTED_EDGE ( 'NONE', *, *, #3268, .F. ) ;
#2437=CARTESIAN_POINT ( 'NONE',  ( -12.32411137850303184, 36.71650635094619730, 80.00000000000000000 ) ) ;
#2444=DIRECTION ( 'NONE',  ( -0.8660254037844377084, 0.5000000000000015543, 0.000000000000000000 ) ) ;
#2446=VERTEX_POINT ( 'NONE', #4507 ) ;
#2450=ORIENTED_EDGE ( 'NONE', *, *, #6316, .T. ) ;
#2463=ORIENTED_EDGE ( 'NONE', *, *, #7704, .T. ) ;
#2473=CARTESIAN_POINT ( 'NONE',  ( 4.025725221640849227, 21.46474596215575659, 79.50000000000000000 ) ) ;
#2477=VECTOR ( 'NONE', #6418, 1000.000000000000000 ) ;
#2480=CARTESIAN_POINT ( 'NONE',  ( -0.9407811293054709756, 40.00000000000008527, 79.50000000000000000 ) ) ;
#2481=CARTESIAN_POINT ( 'NONE',  ( -1.024114462617946808, 43.00000000000008527, 80.00000048127353125 ) ) ;
#2488=CARTESIAN_POINT ( 'NONE',  ( -7.906085446029433861, 41.13124826485289276, 80.00000000000000000 ) ) ;
#2495=ORIENTED_EDGE ( 'NONE', *, *, #5948, .F. ) ;
#2496=EDGE_CURVE ( 'NONE', #4895, #7265, #9751, .T. ) ;
#2504=VECTOR ( 'NONE', #1833, 1000.000000000000000 ) ;
#2509=CARTESIAN_POINT ( 'NONE',  ( 0.000000000000000000, 0.000000000000000000, 79.50000000000000000 ) ) ;
#2511=AXIS2_PLACEMENT_3D ( 'NONE', #11634, #3083, #1094 ) ;
#2512=EDGE_CURVE ( 'NONE', #12341, #7550, #10167, .T. ) ;
#2522=VERTEX_POINT ( 'NONE', #5514 ) ;
#2524=LINE ( 'NONE', #1586, #6707 ) ;
#2535=CARTESIAN_POINT ( 'NONE',  ( 11.80921887069467324, 30.25000000000018474, 79.50000000000000000 ) ) ;
#2541=CARTESIAN_POINT ( 'NONE',  ( 4.025725221640669815, 38.53525403784453118, 79.50000000000000000 ) ) ;
#2544=FACE_OUTER_BOUND ( 'NONE', #8232, .T. ) ;
#2545=FACE_OUTER_BOUND ( 'NONE', #2876, .T. ) ;
#2547=ORIENTED_EDGE ( 'NONE', *, *, #1079, .F. ) ;
#2550=ADVANCED_FACE ( 'NONE', ( #11116 ), #3570, .T. ) ;
#2551=CARTESIAN_POINT ( 'NONE',  ( 0.000000000000000000, 0.000000000000000000, 79.50000000000000000 ) ) ;
#2564=PLANE ( 'NONE',  #6000 ) ;
#2567=EDGE_CURVE ( 'NONE', #1960, #3092, #8602, .T. ) ;
#2569=ADVANCED_FACE ( 'NONE', ( #5814 ), #2068, .T. ) ;
#2572=CARTESIAN_POINT ( 'NONE',  ( -12.32411137850302119, 23.28349364905396612, 80.00000000000000000 ) ) ;
#2574=DIRECTION ( 'NONE',  ( 0.8660254037844420383, 0.4999999999999942824, 0.000000000000000000 ) ) ;
#2575=LINE ( 'NONE', #9414, #5496 ) ;
#2586=VECTOR ( 'NONE', #6126, 1000.000000000000000 ) ;
#2587=DIRECTION ( 'NONE',  ( -1.000000000000000000, 6.938893903907222067E-15, 0.000000000000000000 ) ) ;
#2589=CARTESIAN_POINT ( 'NONE',  ( 9.942549119892413856, 23.28349364905404428, 80.00000000000000000 ) ) ;
#2596=ADVANCED_FACE ( 'NONE', ( #7556 ), #4940, .F. ) ;
#2606=CARTESIAN_POINT ( 'NONE',  ( -12.44911137850311000, 23.50000000000024158, 80.00000000000000000 ) ) ;
#2608=LINE ( 'NONE', #9137, #2477 ) ;
#2609=DIRECTION ( 'NONE',  ( -0.4999999999999942268, 0.8660254037844419273, 0.000000000000000000 ) ) ;
#2611=CARTESIAN_POINT ( 'NONE',  ( -14.19078112930532853, 30.25000000000008882, 79.50000000000000000 ) ) ;
#2614=EDGE_CURVE ( 'NONE', #5368, #5570, #8538, .T. ) ;
#2619=DIRECTION ( 'NONE',  ( 0.8660254037844397068, 0.4999999999999981681, 0.000000000000000000 ) ) ;
#2626=FACE_OUTER_BOUND ( 'NONE', #678, .T. ) ;
#2641=VECTOR ( 'NONE', #10061, 1000.000000000000000 ) ;
#2646=CARTESIAN_POINT ( 'NONE',  ( -1.440781129305282571, 17.00000000000009592, 80.00000000000000000 ) ) ;
#2648=EDGE_CURVE ( 'NONE', #4148, #7445, #12302, .T. ) ;
#2651=CARTESIAN_POINT ( 'NONE',  ( -1.440781129305471087, 40.00000000000008527, 80.00000000000000000 ) ) ;
#2652=DIRECTION ( 'NONE',  ( 0.000000000000000000, -1.000000000000000000, 0.000000000000000000 ) ) ;
#2659=CARTESIAN_POINT ( 'NONE',  ( -0.9407811293054709756, 43.00000000000008527, 79.50000000000000000 ) ) ;
#2664=CARTESIAN_POINT ( 'NONE',  ( 0.000000000000000000, 0.000000000000000000, 79.50000000000000000 ) ) ;
#2672=VECTOR ( 'NONE', #349, 1000.000000000000114 ) ;
#2689=EDGE_CURVE ( 'NONE', #3929, #8835, #3749, .T. ) ;
#2690=DIRECTION ( 'NONE',  ( -0.000000000000000000, -0.000000000000000000, 1.000000000000000000 ) ) ;
#2692=VECTOR ( 'NONE', #7887, 1000.000000000000114 ) ;
#2711=ORIENTED_EDGE ( 'NONE', *, *, #953, .T. ) ;
#2712=CARTESIAN_POINT ( 'NONE',  ( -7.473072744137207124, 41.38124826485288565, 80.00000000000000000 ) ) ;
#2716=CARTESIAN_POINT ( 'NONE',  ( -14.19078112930533209, 29.75000000000008882, 80.00000000000000000 ) ) ;
#2717=DIRECTION ( 'NONE',  ( -1.000000000000000000, 3.469446951953611033E-15, 0.000000000000000000 ) ) ;
#2719=EDGE_CURVE ( 'NONE', #5158, #590, #9658, .T. ) ;
#2723=CARTESIAN_POINT ( 'NONE',  ( -7.907287480251413925, 18.86666975080236597, 80.00000000000000000 ) ) ;
#2725=CARTESIAN_POINT ( 'NONE',  ( -1.190781129305471087, 30.00000000000008882, 80.00000000000000000 ) ) ;
#2747=VERTEX_POINT ( 'NONE', #313 ) ;
#2750=ORIENTED_EDGE ( 'NONE', *, *, #1431, .F. ) ;
#2756=LINE ( 'NONE', #9168, #4692 ) ;
#2757=ORIENTED_EDGE ( 'NONE', *, *, #4392, .T. ) ;
#2769=CARTESIAN_POINT ( 'NONE',  ( 13.80921887069452758, 30.00000000000009237, 80.00000000000000000 ) ) ;
#2786=VERTEX_POINT ( 'NONE', #6055 ) ;
#2807=DIRECTION ( 'NONE',  ( -0.000000000000000000, -1.000000000000000000, 0.000000000000000000 ) ) ;
#2808=AXIS2_PLACEMENT_3D ( 'NONE', #9218, #9469, #12296 ) ;
#2819=EDGE_CURVE ( 'NONE', #11587, #7445, #10029, .T. ) ;
#2823=DIRECTION ( 'NONE',  ( 1.000000000000000000, 0.000000000000000000, 0.000000000000000000 ) ) ;
#2828=AXIS2_PLACEMENT_3D ( 'NONE', #1968, #3774, #2840 ) ;
#2834=CARTESIAN_POINT ( 'NONE',  ( -9.976035167149731819, 34.78349364905394481, 79.50000000000000000 ) ) ;
#2840=DIRECTION ( 'NONE',  ( 0.4999999999999985567, -0.8660254037844394848, 0.000000000000000000 ) ) ;
#2842=VERTEX_POINT ( 'NONE', #6301 ) ;
#2848=DIRECTION ( 'NONE',  ( -1.040834085586083310E-14, -1.000000000000000000, 0.000000000000000000 ) ) ;
#2849=ORIENTED_EDGE ( 'NONE', *, *, #11264, .T. ) ;
#2850=DIRECTION ( 'NONE',  ( -0.4999999999999933387, 0.8660254037844424824, 0.000000000000000000 ) ) ;
#2852=CARTESIAN_POINT ( 'NONE',  ( -12.57411137850301763, 23.71650635094618664, 80.00000000000000000 ) ) ;
#2855=ORIENTED_EDGE ( 'NONE', *, *, #10409, .F. ) ;
#2871=ORIENTED_EDGE ( 'NONE', *, *, #10993, .F. ) ;
#2876=EDGE_LOOP ( 'NONE', ( #9275, #4841, #9522, #3365 ) ) ;
#2878=CARTESIAN_POINT ( 'NONE',  ( -12.57411137850301763, 23.71650635094618664, 80.00000000000000000 ) ) ;
#2879=AXIS2_PLACEMENT_3D ( 'NONE', #7305, #9337, #879 ) ;
#2880=VERTEX_POINT ( 'NONE', #9147 ) ;
#2885=CARTESIAN_POINT ( 'NONE',  ( 10.19254911989230727, 36.28349364905406560, 80.00000000000000000 ) ) ;
#2897=CARTESIAN_POINT ( 'NONE',  ( -7.907287480251421030, 41.13333024919781167, 79.50000000000000000 ) ) ;
#2911=DIRECTION ( 'NONE',  ( 1.000000000000000000, -1.040834085586083310E-14, 0.000000000000000000 ) ) ;
#2914=DIRECTION ( 'NONE',  ( 0.4999999999999985012, -0.8660254037844394848, 0.000000000000000000 ) ) ;
#2917=LINE ( 'NONE', #5847, #11473 ) ;
#2920=EDGE_CURVE ( 'NONE', #8405, #4965, #4486, .T. ) ;
#2926=VERTEX_POINT ( 'NONE', #12040 ) ;
#2942=ORIENTED_EDGE ( 'NONE', *, *, #3703, .F. ) ;
#2949=CARTESIAN_POINT ( 'NONE',  ( -1.440781129305261477, 20.00000000000009592, 79.50000000000000000 ) ) ;
#2950=PLANE ( 'NONE',  #11697 ) ;
#2964=PRESENTATION_STYLE_ASSIGNMENT (( #4902 ) ) ;
#2973=PLANE ( 'NONE',  #3776 ) ;
#2976=DIRECTION ( 'NONE',  ( -0.8660254037844398178, -0.4999999999999977796, 0.000000000000000000 ) ) ;
#2982=AXIS2_PLACEMENT_3D ( 'NONE', #10327, #6353, #9325 ) ;
#2992=DIRECTION ( 'NONE',  ( 0.8660254037844331565, -0.5000000000000095479, 0.000000000000000000 ) ) ;
#2995=DIRECTION ( 'NONE',  ( 0.5000000000000001110, 0.8660254037844387076, 0.000000000000000000 ) ) ;
#2996=DIRECTION ( 'NONE',  ( -0.4999999999999942268, 0.8660254037844419273, 0.000000000000000000 ) ) ;
#3012=CARTESIAN_POINT ( 'NONE',  ( -14.19078112930533209, 29.75000000000008882, 79.50000000000000000 ) ) ;
#3013=CARTESIAN_POINT ( 'NONE',  ( 5.092712519748452848, 41.38333024919784719, 79.50000000000000000 ) ) ;
#3015=CARTESIAN_POINT ( 'NONE',  ( -1.190781129305471087, 30.00000000000008882, 80.00000000000000000 ) ) ;
#3016=PLANE ( 'NONE',  #7168 ) ;
#3020=ORIENTED_EDGE ( 'NONE', *, *, #12206, .T. ) ;
#3024=VECTOR ( 'NONE', #4583, 1000.000000000000000 ) ;
#3039=VERTEX_POINT ( 'NONE', #4669 ) ;
#3046=EDGE_CURVE ( 'NONE', #4833, #10602, #4728, .T. ) ;
#3051=ORIENTED_EDGE ( 'NONE', *, *, #200, .F. ) ;
#3058=CARTESIAN_POINT ( 'NONE',  ( -5.974274778359173865, 21.21474596215567487, 79.50000000000000000 ) ) ;
#3059=ORIENTED_EDGE ( 'NONE', *, *, #681, .T. ) ;
#3061=AXIS2_PLACEMENT_3D ( 'NONE', #8815, #7143, #6091 ) ;
#3065=LINE ( 'NONE', #6745, #9242 ) ;
#3068=PLANE ( 'NONE',  #11071 ) ;
#3072=EDGE_CURVE ( 'NONE', #11346, #3399, #3927, .T. ) ;
#3077=CARTESIAN_POINT ( 'NONE',  ( -7.907287480251413925, 18.86666975080236597, 79.50000000000000000 ) ) ;
#3082=LINE ( 'NONE', #8866, #8432 ) ;
#3083=DIRECTION ( 'NONE',  ( -0.000000000000000000, -0.000000000000000000, -1.000000000000000000 ) ) ;
#3087=SURFACE_STYLE_FILL_AREA ( #5899 ) ;
#3091=ORIENTED_EDGE ( 'NONE', *, *, #9038, .F. ) ;
#3092=VERTEX_POINT ( 'NONE', #10399 ) ;
#3094=DIRECTION ( 'NONE',  ( 0.8660254037844399289, 0.4999999999999977796, 0.000000000000000000 ) ) ;
#3098=PLANE ( 'NONE',  #11873 ) ;
#3101=B_SPLINE_CURVE_WITH_KNOTS ( 'NONE', 3,
 ( #2151, #9741, #6708, #5958 ),
 .UNSPECIFIED., .F., .F.,
 ( 4, 4 ),
 ( 0.0002502309401076680852, 0.0005002309401076784987 ),
 .UNSPECIFIED. ) ;
#3103=EDGE_CURVE ( 'NONE', #11846, #1468, #171, .T. ) ;
#3109=ORIENTED_EDGE ( 'NONE', *, *, #2496, .T. ) ;
#3111=CARTESIAN_POINT ( 'NONE',  ( 9.942549119892413856, 23.28349364905404428, 79.50000000000000000 ) ) ;
#3117=VECTOR ( 'NONE', #6095, 1000.000000000000114 ) ;
#3120=ORIENTED_EDGE ( 'NONE', *, *, #6635, .T. ) ;
#3123=AXIS2_PLACEMENT_3D ( 'NONE', #8484, #6815, #10612 ) ;
#3124=ORIENTED_EDGE ( 'NONE', *, *, #2648, .F. ) ;
#3125=DIRECTION ( 'NONE',  ( -0.000000000000000000, -0.000000000000000000, 1.000000000000000000 ) ) ;
#3132=ADVANCED_FACE ( 'NONE', ( #9517 ), #8462, .T. ) ;
#3141=EDGE_CURVE ( 'NONE', #9412, #3881, #12286, .T. ) ;
#3148=DIRECTION ( 'NONE',  ( 0.5000000000000038858, 0.8660254037844363761, 0.000000000000000000 ) ) ;
#3154=EDGE_CURVE ( 'NONE', #3039, #3929, #7659, .T. ) ;
#3156=VECTOR ( 'NONE', #5587, 1000.000000000000000 ) ;
#3157=CARTESIAN_POINT ( 'NONE',  ( -1.190781129305471087, 30.00000000000008882, 80.00000000000000000 ) ) ;
#3162=EDGE_LOOP ( 'NONE', ( #2022, #11244, #6013, #9011, #11184 ) ) ;
#3164=EDGE_CURVE ( 'NONE', #5158, #2274, #46, .T. ) ;
#3165=EDGE_LOOP ( 'NONE', ( #9598, #8663, #9347, #10099, #10565 ) ) ;
#3166=CARTESIAN_POINT ( 'NONE',  ( -12.57411137850303540, 36.28349364905398033, 79.50000000000000000 ) ) ;
#3168=ORIENTED_EDGE ( 'NONE', *, *, #1176, .T. ) ;
#3175=DIRECTION ( 'NONE',  ( -0.000000000000000000, -0.000000000000000000, 1.000000000000000000 ) ) ;
#3190=CARTESIAN_POINT ( 'NONE',  ( -0.9407811293052825707, 17.00000000000008882, 80.00000000000000000 ) ) ;
#3196=AXIS2_PLACEMENT_3D ( 'NONE', #7951, #3289, #9823 ) ;
#3198=CARTESIAN_POINT ( 'NONE',  ( -7.690781129305409358, 41.25833024919774772, 80.00000000000000000 ) ) ;
#3202=ORIENTED_EDGE ( 'NONE', *, *, #10324, .F. ) ;
#3205=VERTEX_POINT ( 'NONE', #11891 ) ;
#3208=VERTEX_POINT ( 'NONE', #11659 ) ;
#3209=DIRECTION ( 'NONE',  ( -0.000000000000000000, -0.000000000000000000, 1.000000000000000000 ) ) ;
#3239=ORIENTED_EDGE ( 'NONE', *, *, #1370, .F. ) ;
#3260=EDGE_LOOP ( 'NONE', ( #3091, #2073, #3433, #7906, #2871 ) ) ;
#3261=DIRECTION ( 'NONE',  ( 0.000000000000000000, -1.000000000000000000, 0.000000000000000000 ) ) ;
#3264=DIRECTION ( 'NONE',  ( 1.000000000000000000, -1.387778780781445676E-14, 0.000000000000000000 ) ) ;
#3268=EDGE_CURVE ( 'NONE', #893, #4148, #8996, .T. ) ;
#3274=ORIENTED_EDGE ( 'NONE', *, *, #3662, .T. ) ;
#3275=EDGE_CURVE ( 'NONE', #2274, #11587, #7840, .T. ) ;
#3288=ORIENTED_EDGE ( 'NONE', *, *, #2648, .T. ) ;
#3289=DIRECTION ( 'NONE',  ( -0.4999999999999977796, 0.8660254037844399289, 0.000000000000000000 ) ) ;
#3292=ORIENTED_EDGE ( 'NONE', *, *, #7210, .T. ) ;
#3300=DIRECTION ( 'NONE',  ( 0.4999999999999985012, 0.8660254037844394848, 0.000000000000000000 ) ) ;
#3302=ORIENTED_EDGE ( 'NONE', *, *, #927, .T. ) ;
#3312=VECTOR ( 'NONE', #1465, 1000.000000000000000 ) ;
#3320=ORIENTED_EDGE ( 'NONE', *, *, #8449, .F. ) ;
#3321=LINE ( 'NONE', #7060, #2586 ) ;
#3337=ORIENTED_EDGE ( 'NONE', *, *, #10324, .T. ) ;
#3341=DIRECTION ( 'NONE',  ( -6.938893903907222067E-15, -1.000000000000000000, 0.000000000000000000 ) ) ;
#3347=CARTESIAN_POINT ( 'NONE',  ( -12.57411137850303540, 36.28349364905398033, 80.00000000000000000 ) ) ;
#3350=LINE ( 'NONE', #12143, #10779 ) ;
#3352=EDGE_CURVE ( 'NONE', #5980, #1372, #11131, .T. ) ;
#3354=CARTESIAN_POINT ( 'NONE',  ( 10.19254911989241386, 23.71650635094626836, 79.50000000000000000 ) ) ;
#3365=ORIENTED_EDGE ( 'NONE', *, *, #7691, .F. ) ;
#3374=ORIENTED_EDGE ( 'NONE', *, *, #1598, .T. ) ;
#3375=CARTESIAN_POINT ( 'NONE',  ( 10.19254911989241386, 23.71650635094626836, 79.50000000000000000 ) ) ;
#3377=ORIENTED_EDGE ( 'NONE', *, *, #7141, .F. ) ;
#3378=DIRECTION ( 'NONE',  ( 0.000000000000000000, 0.000000000000000000, 1.000000000000000000 ) ) ;
#3387=EDGE_CURVE ( 'NONE', #7990, #2747, #6393, .T. ) ;
#3389=CARTESIAN_POINT ( 'NONE',  ( -7.907287480251421030, 41.13333024919781167, 79.50000000000000000 ) ) ;
#3390=FACE_OUTER_BOUND ( 'NONE', #4413, .T. ) ;
#3398=PLANE ( 'NONE',  #11169 ) ;
#3399=VERTEX_POINT ( 'NONE', #2834 ) ;
#3404=VECTOR ( 'NONE', #4142, 1000.000000000000000 ) ;
#3406=CARTESIAN_POINT ( 'NONE',  ( -6.407287480251391720, 21.46474596215567487, 79.50000000000000000 ) ) ;
#3413=VECTOR ( 'NONE', #12115, 1000.000000000000227 ) ;
#3414=CARTESIAN_POINT ( 'NONE',  ( 5.525725221640833240, 18.86666975080242992, 79.50000000000000000 ) ) ;
#3417=CARTESIAN_POINT ( 'NONE',  ( -14.18837706086142703, 30.25000000000008882, 80.00000000000000000 ) ) ;
#3418=DIRECTION ( 'NONE',  ( 0.8660254037844434816, 0.4999999999999913958, 0.000000000000000000 ) ) ;
#3422=VERTEX_POINT ( 'NONE', #6639 ) ;
#3433=ORIENTED_EDGE ( 'NONE', *, *, #10409, .T. ) ;
#3440=VERTEX_POINT ( 'NONE', #9244 ) ;
#3452=CARTESIAN_POINT ( 'NONE',  ( -1.440781129305261477, 20.00000000000009592, 79.50000000000000000 ) ) ;
#3454=EDGE_CURVE ( 'NONE', #867, #434, #8685, .T. ) ;
#3482=CARTESIAN_POINT ( 'NONE',  ( -7.835118696620823719, 18.82500308414615731, 80.00000048127353125 ) ) ;
#3484=ORIENTED_EDGE ( 'NONE', *, *, #1288, .F. ) ;
#3486=DIRECTION ( 'NONE',  ( 0.8660254037844394848, 0.4999999999999985567, 0.000000000000000000 ) ) ;
#3490=PLANE ( 'NONE',  #6172 ) ;
#3499=ORIENTED_EDGE ( 'NONE', *, *, #4666, .T. ) ;
#3500=ADVANCED_FACE ( 'NONE', ( #8802 ), #5833, .F. ) ;
#3506=DIRECTION ( 'NONE',  ( 3.469446951953611033E-15, 1.000000000000000000, 0.000000000000000000 ) ) ;
#3508=CARTESIAN_POINT ( 'NONE',  ( 7.344472908538985045, 35.21650635094629678, 79.50000000000000000 ) ) ;
#3512=ORIENTED_EDGE ( 'NONE', *, *, #596, .T. ) ;
#3513=ADVANCED_FACE ( 'NONE', ( #271 ), #82, .T. ) ;
#3514=DIRECTION ( 'NONE',  ( 0.000000000000000000, 0.000000000000000000, 1.000000000000000000 ) ) ;
#3516=DIRECTION ( 'NONE',  ( 0.8660254037844434816, 0.4999999999999913958, 0.000000000000000000 ) ) ;
#3525=VECTOR ( 'NONE', #1204, 1000.000000000000114 ) ;
#3537=EDGE_LOOP ( 'NONE', ( #5793, #9643, #8350, #7032, #6262 ) ) ;
#3539=DIRECTION ( 'NONE',  ( -0.8660254037844403729, -0.4999999999999970024, 0.000000000000000000 ) ) ;
#3545=CARTESIAN_POINT ( 'NONE',  ( -12.53244471184681075, 23.64433756731560266, 80.00000048127353125 ) ) ;
#3551=AXIS2_PLACEMENT_3D ( 'NONE', #11475, #3861, #2053 ) ;
#3570=PLANE ( 'NONE',  #9533 ) ;
#3573=DIRECTION ( 'NONE',  ( -0.4999999999999942268, 0.8660254037844419273, 0.000000000000000000 ) ) ;
#3577=CARTESIAN_POINT ( 'NONE',  ( -5.974274778359173865, 21.21474596215567487, 80.00000000000000000 ) ) ;
#3589=LINE ( 'NONE', #4458, #8976 ) ;
#3591=PLANE ( 'NONE',  #11484 ) ;
#3597=DIRECTION ( 'NONE',  ( 0.8660254037844397068, 0.4999999999999981681, 0.000000000000000000 ) ) ;
#3611=LINE ( 'NONE', #9204, #4174 ) ;
#3619=CARTESIAN_POINT ( 'NONE',  ( 3.592712519748626931, 21.21474596215575659, 79.50000000000000000 ) ) ;
#3628=LINE ( 'NONE', #9160, #4005 ) ;
#3635=DIRECTION ( 'NONE',  ( 0.000000000000000000, 0.000000000000000000, 1.000000000000000000 ) ) ;
#3643=VERTEX_POINT ( 'NONE', #4567 ) ;
#3644=ORIENTED_EDGE ( 'NONE', *, *, #449, .F. ) ;
#3648=CARTESIAN_POINT ( 'NONE',  ( 11.80921887069467324, 30.25000000000018474, 79.50000000000000000 ) ) ;
#3650=LINE ( 'NONE', #9247, #3024 ) ;
#3654=CARTESIAN_POINT ( 'NONE',  ( 5.092712519748611832, 18.61666975080242992, 79.50000000000000000 ) ) ;
#3656=VECTOR ( 'NONE', #2850, 1000.000000000000114 ) ;
#3659=CARTESIAN_POINT ( 'NONE',  ( -7.474274778359198734, 41.38333024919781167, 80.00000000000000000 ) ) ;
#3662=EDGE_CURVE ( 'NONE', #10032, #8236, #5897, .T. ) ;
#3670=DIRECTION ( 'NONE',  ( -6.938893903907222067E-15, -1.000000000000000000, 0.000000000000000000 ) ) ;
#3674=PRODUCT_DEFINITION ( 'UNKNOWN', '', #11531, #10743 ) ;
#3692=CARTESIAN_POINT ( 'NONE',  ( 13.80921887069452758, 30.00000000000009237, 65.00000000000000000 ) ) ;
#3694=ORIENTED_EDGE ( 'NONE', *, *, #5318, .F. ) ;
#3703=EDGE_CURVE ( 'NONE', #4222, #11096, #2756, .T. ) ;
#3705=EDGE_CURVE ( 'NONE', #938, #7550, #2575, .T. ) ;
#3708=CARTESIAN_POINT ( 'NONE',  ( -0.9407811293052825707, 17.00000000000008882, 80.00000000000000000 ) ) ;
#3716=VECTOR ( 'NONE', #4447, 1000.000000000000000 ) ;
#3724=CARTESIAN_POINT ( 'NONE',  ( -1.440781129305282571, 17.00000000000009592, 79.50000000000000000 ) ) ;
#3731=ADVANCED_FACE ( 'NONE', ( #9479 ), #3068, .F. ) ;
#3733=DIRECTION ( 'NONE',  ( 0.8660254037844331565, -0.5000000000000095479, 0.000000000000000000 ) ) ;
#3739=CARTESIAN_POINT ( 'NONE',  ( 5.525725221640672480, 41.13333024919784719, 80.00000000000000000 ) ) ;
#3746=LINE ( 'NONE', #7496, #1416 ) ;
#3747=EDGE_LOOP ( 'NONE', ( #6322, #10090, #5519, #9965, #4660 ) ) ;
#3749=LINE ( 'NONE', #11551, #6762 ) ;
#3755=VERTEX_POINT ( 'NONE', #8791 ) ;
#3759=LINE ( 'NONE', #2885, #4594 ) ;
#3766=DIRECTION ( 'NONE',  ( -0.8660254037844377084, 0.5000000000000015543, 0.000000000000000000 ) ) ;
#3771=VECTOR ( 'NONE', #10483, 1000.000000000000114 ) ;
#3774=DIRECTION ( 'NONE',  ( -0.8660254037844394848, -0.4999999999999985567, 0.000000000000000000 ) ) ;
#3776=AXIS2_PLACEMENT_3D ( 'NONE', #10386, #2848, #2911 ) ;
#3791=CARTESIAN_POINT ( 'NONE',  ( -1.190781129305471087, 30.00000000000008882, 80.00000000000000000 ) ) ;
#3804=ADVANCED_FACE ( 'NONE', ( #2072 ), #6, .F. ) ;
#3814=ADVANCED_FACE ( 'NONE', ( #4944 ), #10545, .T. ) ;
#3816=ORIENTED_EDGE ( 'NONE', *, *, #4910, .T. ) ;
#3819=ORIENTED_EDGE ( 'NONE', *, *, #10882, .T. ) ;
#3821=DIRECTION ( 'NONE',  ( 0.8660254037844331565, -0.5000000000000095479, 0.000000000000000000 ) ) ;
#3824=CARTESIAN_POINT ( 'NONE',  ( -14.19078112930533209, 29.75000000000008882, 79.50000000000000000 ) ) ;
#3825=DIRECTION ( 'NONE',  ( -0.000000000000000000, -0.000000000000000000, 1.000000000000000000 ) ) ;
#3830=ORIENTED_EDGE ( 'NONE', *, *, #5344, .F. ) ;
#3835=DIRECTION ( 'NONE',  ( 1.000000000000000000, -1.040834085586083310E-14, 0.000000000000000000 ) ) ;
#3839=DIRECTION ( 'NONE',  ( 0.000000000000000000, 0.000000000000000000, 1.000000000000000000 ) ) ;
#3844=EDGE_CURVE ( 'NONE', #4861, #4898, #7974, .T. ) ;
#3852=AXIS2_PLACEMENT_3D ( 'NONE', #3157, #344, #11006 ) ;
#3856=CARTESIAN_POINT ( 'NONE',  ( 9.942549119892413856, 23.28349364905404428, 80.00000000000000000 ) ) ;
#3857=AXIS2_PLACEMENT_3D ( 'NONE', #9488, #972, #4762 ) ;
#3861=DIRECTION ( 'NONE',  ( -0.4999999999999985567, 0.8660254037844394848, 0.000000000000000000 ) ) ;
#3869=CARTESIAN_POINT ( 'NONE',  ( -0.9407811293054709756, 40.00000000000008527, 80.00000000000000000 ) ) ;
#3875=PLANE ( 'NONE',  #9514 ) ;
#3876=ORIENTED_EDGE ( 'NONE', *, *, #11312, .F. ) ;
#3881=VERTEX_POINT ( 'NONE', #9909 ) ;
#3882=CIRCLE ( 'NONE', #1696, 12.99999999999999822 ) ;
#3889=DIRECTION ( 'NONE',  ( -0.000000000000000000, -0.000000000000000000, 1.000000000000000000 ) ) ;
#3895=( NAMED_UNIT ( * ) PLANE_ANGLE_UNIT ( ) SI_UNIT ( $, .RADIAN. ) );
#3901=ORIENTED_EDGE ( 'NONE', *, *, #11948, .F. ) ;
#3902=FACE_OUTER_BOUND ( 'NONE', #3747, .T. ) ;
#3905=SURFACE_SIDE_STYLE ('',( #3087 ) ) ;
#3912=VECTOR ( 'NONE', #8132, 1000.000000000000000 ) ;
#3913=LINE ( 'NONE', #7470, #11466 ) ;
#3915=FACE_OUTER_BOUND ( 'NONE', #2048, .T. ) ;
#3922=VERTEX_POINT ( 'NONE', #1444 ) ;
#3927=LINE ( 'NONE', #1929, #8108 ) ;
#3929=VERTEX_POINT ( 'NONE', #5249 ) ;
#3930=LINE ( 'NONE', #8775, #11854 ) ;
#3931=DIRECTION ( 'NONE',  ( -0.4999999999999985567, -0.8660254037844394848, 0.000000000000000000 ) ) ;
#3935=LINE ( 'NONE', #9776, #7197 ) ;
#3936=ORIENTED_EDGE ( 'NONE', *, *, #1598, .F. ) ;
#3949=FACE_OUTER_BOUND ( 'NONE', #7911, .T. ) ;
#3951=DIRECTION ( 'NONE',  ( -0.4999999999999942268, 0.8660254037844419273, 0.000000000000000000 ) ) ;
#3956=( NAMED_UNIT ( * ) SI_UNIT ( $, .STERADIAN. ) SOLID_ANGLE_UNIT ( ) );
#3987=EDGE_LOOP ( 'NONE', ( #10843, #4710, #9224, #4257, #7764 ) ) ;
#4004=AXIS2_PLACEMENT_3D ( 'NONE', #10613, #10676, #5887 ) ;
#4005=VECTOR ( 'NONE', #2690, 1000.000000000000000 ) ;
#4015=ORIENTED_EDGE ( 'NONE', *, *, #1431, .T. ) ;
#4021=VECTOR ( 'NONE', #7145, 1000.000000000000000 ) ;
#4023=DIRECTION ( 'NONE',  ( -0.4999999999999933387, 0.8660254037844424824, 0.000000000000000000 ) ) ;
#4036=B_SPLINE_CURVE_WITH_KNOTS ( 'NONE', 3,
 ( #2606, #12214, #3545, #2852 ),
 .UNSPECIFIED., .F., .F.,
 ( 4, 4 ),
 ( 0.0002502309401078630247, 0.0005002309401076750293 ),
 .UNSPECIFIED. ) ;
#4050=DIRECTION ( 'NONE',  ( 1.000000000000000000, 0.000000000000000000, 0.000000000000000000 ) ) ;
#4057=ORIENTED_EDGE ( 'NONE', *, *, #9903, .T. ) ;
#4061=ADVANCED_FACE ( 'NONE', ( #12044 ), #692, .T. ) ;
#4063=CARTESIAN_POINT ( 'NONE',  ( 7.344472908538985045, 35.21650635094629678, 79.50000000000000000 ) ) ;
#4072=CARTESIAN_POINT ( 'NONE',  ( 10.19254911989241386, 23.71650635094626836, 79.50000000000000000 ) ) ;
#4075=FACE_OUTER_BOUND ( 'NONE', #1348, .T. ) ;
#4088=EDGE_CURVE ( 'NONE', #3422, #65, #4469, .T. ) ;
#4089=EDGE_CURVE ( 'NONE', #12119, #10896, #3930, .T. ) ;
#4097=DIRECTION ( 'NONE',  ( 0.000000000000000000, 0.000000000000000000, 1.000000000000000000 ) ) ;
#4105=AXIS2_PLACEMENT_3D ( 'NONE', #4864, #8651, #3931 ) ;
#4107=DIRECTION ( 'NONE',  ( -0.000000000000000000, -0.000000000000000000, -1.000000000000000000 ) ) ;
#4110=LINE ( 'NONE', #240, #4298 ) ;
#4113=AXIS2_PLACEMENT_3D ( 'NONE', #9930, #3148, #9050 ) ;
#4120=ORIENTED_EDGE ( 'NONE', *, *, #3352, .T. ) ;
#4123=ORIENTED_EDGE ( 'NONE', *, *, #7393, .T. ) ;
#4133=ORIENTED_EDGE ( 'NONE', *, *, #5258, .F. ) ;
#4137=CARTESIAN_POINT ( 'NONE',  ( 5.524523187418616033, 41.13124826485281460, 80.00000000000000000 ) ) ;
#4141=CARTESIAN_POINT ( 'NONE',  ( 5.237050087044693214, 18.70000308413499823, 80.00000000000000000 ) ) ;
#4142=DIRECTION ( 'NONE',  ( -0.000000000000000000, -0.000000000000000000, 1.000000000000000000 ) ) ;
#4147=( GEOMETRIC_REPRESENTATION_CONTEXT ( 3 ) GLOBAL_UNCERTAINTY_ASSIGNED_CONTEXT ( ( #11394 ) ) GLOBAL_UNIT_ASSIGNED_CONTEXT ( ( #967, #3895, #6821 ) ) REPRESENTATION_CONTEXT ( 'NONE', 'WORKASPACE' ) );
#4148=VERTEX_POINT ( 'NONE', #11479 ) ;
#4151=FACE_OUTER_BOUND ( 'NONE', #667, .T. ) ;
#4174=VECTOR ( 'NONE', #7419, 1000.000000000000000 ) ;
#4188=VECTOR ( 'NONE', #9316, 1000.000000000000114 ) ;
#4195=ADVANCED_FACE ( 'NONE', ( #2419 ), #10775, .F. ) ;
#4199=ORIENTED_EDGE ( 'NONE', *, *, #6254, .F. ) ;
#4200=DIRECTION ( 'NONE',  ( -1.000000000000000000, 3.469446951953611033E-15, 0.000000000000000000 ) ) ;
#4205=DIRECTION ( 'NONE',  ( 6.938893903907222067E-15, 1.000000000000000000, 0.000000000000000000 ) ) ;
#4219=SHAPE_DEFINITION_REPRESENTATION ( #7872, #12244 ) ;
#4222=VERTEX_POINT ( 'NONE', #6974 ) ;
#4241=FACE_OUTER_BOUND ( 'NONE', #10331, .T. ) ;
#4243=ORIENTED_EDGE ( 'NONE', *, *, #9744, .T. ) ;
#4244=FACE_OUTER_BOUND ( 'NONE', #4272, .T. ) ;
#4246=DIRECTION ( 'NONE',  ( -1.000000000000000000, 3.469446951953611033E-15, 0.000000000000000000 ) ) ;
#4247=VECTOR ( 'NONE', #2976, 1000.000000000000114 ) ;
#4248=ORIENTED_EDGE ( 'NONE', *, *, #39, .F. ) ;
#4256=VECTOR ( 'NONE', #2807, 1000.000000000000000 ) ;
#4257=ORIENTED_EDGE ( 'NONE', *, *, #10379, .T. ) ;
#4271=VECTOR ( 'NONE', #2045, 1000.000000000000114 ) ;
#4272=EDGE_LOOP ( 'NONE', ( #10114, #7259, #2067, #3644 ) ) ;
#4275=DIRECTION ( 'NONE',  ( -0.5000000000000036637, -0.8660254037844364872, 0.000000000000000000 ) ) ;
#4278=VECTOR ( 'NONE', #9042, 1000.000000000000000 ) ;
#4287=DIRECTION ( 'NONE',  ( -0.5000000000000001110, -0.8660254037844387076, 0.000000000000000000 ) ) ;
#4288=EDGE_LOOP ( 'NONE', ( #4983, #1979, #8497, #8960 ) ) ;
#4296=ORIENTED_EDGE ( 'NONE', *, *, #10472, .T. ) ;
#4298=VECTOR ( 'NONE', #2992, 1000.000000000000114 ) ;
#4306=ORIENTED_EDGE ( 'NONE', *, *, #2496, .F. ) ;
#4319=ORIENTED_EDGE ( 'NONE', *, *, #6863, .T. ) ;
#4320=LINE ( 'NONE', #8116, #9597 ) ;
#4329=ADVANCED_FACE ( 'NONE', ( #2545 ), #616, .F. ) ;
#4332=CARTESIAN_POINT ( 'NONE',  ( -14.19078112930532853, 30.16666666668764307, 80.00000048127353125 ) ) ;
#4337=B_SPLINE_CURVE_WITH_KNOTS ( 'NONE', 3,
 ( #12079, #7270, #11132, #2589 ),
 .UNSPECIFIED., .F., .F.,
 ( 4, 4 ),
 ( 0.0002502309401078032310, 0.0005002309401076767640 ),
 .UNSPECIFIED. ) ;
#4340=CARTESIAN_POINT ( 'NONE',  ( -5.974274778359230709, 38.78525403784446723, 79.50000000000000000 ) ) ;
#4351=ORIENTED_EDGE ( 'NONE', *, *, #5560, .T. ) ;
#4357=VECTOR ( 'NONE', #2167, 1000.000000000000000 ) ;
#4369=FACE_OUTER_BOUND ( 'NONE', #11067, .T. ) ;
#4381=DIRECTION ( 'NONE',  ( 0.000000000000000000, 0.000000000000000000, -1.000000000000000000 ) ) ;
#4392=EDGE_CURVE ( 'NONE', #2926, #7629, #4792, .T. ) ;
#4402=CARTESIAN_POINT ( 'NONE',  ( -12.57411137850301763, 23.71650635094618664, 80.00000000000000000 ) ) ;
#4411=CARTESIAN_POINT ( 'NONE',  ( -7.690781129305457320, 18.74166975080245834, 80.00000000000000000 ) ) ;
#4413=EDGE_LOOP ( 'NONE', ( #2495, #2393, #8521, #1334, #11816 ) ) ;
#4415=VECTOR ( 'NONE', #4708, 1000.000000000000227 ) ;
#4418=FACE_OUTER_BOUND ( 'NONE', #3537, .T. ) ;
#4425=ORIENTED_EDGE ( 'NONE', *, *, #12198, .T. ) ;
#4431=LINE ( 'NONE', #5314, #10493 ) ;
#4439=CARTESIAN_POINT ( 'NONE',  ( -7.907287480251421030, 41.13333024919781167, 79.50000000000000000 ) ) ;
#4440=ORIENTED_EDGE ( 'NONE', *, *, #11628, .F. ) ;
#4447=DIRECTION ( 'NONE',  ( 0.8660254037844397068, 0.4999999999999981681, 0.000000000000000000 ) ) ;
#4450=ADVANCED_FACE ( 'NONE', ( #10321 ), #9321, .F. ) ;
#4458=CARTESIAN_POINT ( 'NONE',  ( -7.474274778359196070, 18.61666975080236597, 80.00000000000000000 ) ) ;
#4459=CARTESIAN_POINT ( 'NONE',  ( 5.092712519748452848, 41.38333024919784719, 79.50000000000000000 ) ) ;
#4467=LINE ( 'NONE', #8384, #6386 ) ;
#4469=CIRCLE ( 'NONE', #9239, 12.99999999999999822 ) ;
#4474=CARTESIAN_POINT ( 'NONE',  ( -7.762949912955313891, 18.78333641746978699, 80.00000000000000000 ) ) ;
#4480=AXIS2_PLACEMENT_3D ( 'NONE', #6030, #470, #11648 ) ;
#4483=AXIS2_PLACEMENT_3D ( 'NONE', #11417, #10656, #9709 ) ;
#4486=LINE ( 'NONE', #11034, #7124 ) ;
#4491=CARTESIAN_POINT ( 'NONE',  ( -1.440781129305471087, 43.00000000000008527, 79.50000000000000000 ) ) ;
#4503=DIRECTION ( 'NONE',  ( 0.4999999999999985012, -0.8660254037844394848, 0.000000000000000000 ) ) ;
#4507=CARTESIAN_POINT ( 'NONE',  ( -16.19078112930547064, 30.00000000000008882, 78.00000000000000000 ) ) ;
#4508=DIRECTION ( 'NONE',  ( 1.000000000000000000, 0.000000000000000000, -0.000000000000000000 ) ) ;
#4523=LINE ( 'NONE', #2646, #6051 ) ;
#4525=LINE ( 'NONE', #11266, #2641 ) ;
#4533=CARTESIAN_POINT ( 'NONE',  ( 3.592712519748626931, 21.21474596215575659, 80.00000000000000000 ) ) ;
#4549=LINE ( 'NONE', #7364, #9565 ) ;
#4560=B_SPLINE_CURVE_WITH_KNOTS ( 'NONE', 3,
 ( #11829, #7082, #10881, #5462 ),
 .UNSPECIFIED., .F., .F.,
 ( 4, 4 ),
 ( 0.0002502309401077386667, 0.0005002309401076767640 ),
 .UNSPECIFIED. ) ;
#4564=CARTESIAN_POINT ( 'NONE',  ( -1.274114462640252521, 17.00000000000009237, 80.00000000000000000 ) ) ;
#4567=CARTESIAN_POINT ( 'NONE',  ( -12.57411137850301763, 23.71650635094618664, 80.00000000000000000 ) ) ;
#4568=VERTEX_POINT ( 'NONE', #10577 ) ;
#4569=DIRECTION ( 'NONE',  ( -0.000000000000000000, -1.000000000000000000, 0.000000000000000000 ) ) ;
#4570=LINE ( 'NONE', #8365, #6391 ) ;
#4578=B_SPLINE_CURVE_WITH_KNOTS ( 'NONE', 3,
 ( #741, #610, #2481, #5477 ),
 .UNSPECIFIED., .F., .F.,
 ( 4, 4 ),
 ( 0.0009573067811865457882, 0.001207306781186546010 ),
 .UNSPECIFIED. ) ;
#4580=CARTESIAN_POINT ( 'NONE',  ( -7.907287480251413925, 18.86666975080236597, 79.50000000000000000 ) ) ;
#4583=DIRECTION ( 'NONE',  ( -0.000000000000000000, -0.000000000000000000, 1.000000000000000000 ) ) ;
#4587=ORIENTED_EDGE ( 'NONE', *, *, #11781, .F. ) ;
#4589=VECTOR ( 'NONE', #5489, 1000.000000000000000 ) ;
#4594=VECTOR ( 'NONE', #5764, 1000.000000000000114 ) ;
#4595=VECTOR ( 'NONE', #4503, 1000.000000000000114 ) ;
#4600=CARTESIAN_POINT ( 'NONE',  ( 4.025725221640849227, 21.46474596215575659, 80.00000000000000000 ) ) ;
#4602=DIRECTION ( 'NONE',  ( 0.000000000000000000, 0.000000000000000000, 1.000000000000000000 ) ) ;
#4604=ORIENTED_EDGE ( 'NONE', *, *, #5572, .T. ) ;
#4605=DIRECTION ( 'NONE',  ( -0.000000000000000000, -0.000000000000000000, 1.000000000000000000 ) ) ;
#4606=AXIS2_PLACEMENT_3D ( 'NONE', #9725, #5010, #9607 ) ;
#4621=EDGE_CURVE ( 'NONE', #6185, #10487, #8699, .T. ) ;
#4622=LINE ( 'NONE', #5509, #1225 ) ;
#4624=VECTOR ( 'NONE', #9371, 1000.000000000000000 ) ;
#4629=DIRECTION ( 'NONE',  ( -0.5000000000000006661, -0.8660254037844383745, 0.000000000000000000 ) ) ;
#4648=CARTESIAN_POINT ( 'NONE',  ( -7.907287480251421030, 41.13333024919781167, 79.50000000000000000 ) ) ;
#4656=CARTESIAN_POINT ( 'NONE',  ( 8.809218870694669690, 29.75000000000019540, 79.50000000000000000 ) ) ;
#4660=ORIENTED_EDGE ( 'NONE', *, *, #8369, .F. ) ;
#4666=EDGE_CURVE ( 'NONE', #3422, #11988, #6593, .T. ) ;
#4669=CARTESIAN_POINT ( 'NONE',  ( 5.092712519748611832, 18.61666975080242992, 80.00000000000000000 ) ) ;
#4673=ORIENTED_EDGE ( 'NONE', *, *, #7241, .T. ) ;
#4679=FACE_OUTER_BOUND ( 'NONE', #10710, .T. ) ;
#4686=DIRECTION ( 'NONE',  ( 1.000000000000000000, 0.000000000000000000, 0.000000000000000000 ) ) ;
#4687=ORIENTED_EDGE ( 'NONE', *, *, #510, .F. ) ;
#4691=CARTESIAN_POINT ( 'NONE',  ( -0.9407811293052614765, 20.00000000000009237, 80.00000000000000000 ) ) ;
#4692=VECTOR ( 'NONE', #6564, 1000.000000000000000 ) ;
#4698=EDGE_CURVE ( 'NONE', #5363, #11844, #9816, .T. ) ;
#4700=LINE ( 'NONE', #848, #12027 ) ;
#4705=CARTESIAN_POINT ( 'NONE',  ( -14.19078112930532853, 30.25000000000008882, 79.50000000000000000 ) ) ;
#4708=DIRECTION ( 'NONE',  ( -0.8660254037844385966, 0.5000000000000000000, 0.000000000000000000 ) ) ;
#4710=ORIENTED_EDGE ( 'NONE', *, *, #4838, .F. ) ;
#4722=PLANE ( 'NONE',  #7056 ) ;
#4723=DIRECTION ( 'NONE',  ( 0.000000000000000000, 0.000000000000000000, -1.000000000000000000 ) ) ;
#4725=LINE ( 'NONE', #5426, #197 ) ;
#4728=LINE ( 'NONE', #5858, #969 ) ;
#4735=CARTESIAN_POINT ( 'NONE',  ( 11.80921887069467324, 29.75000000000018474, 80.00000000000000000 ) ) ;
#4737=DIRECTION ( 'NONE',  ( -1.000000000000000000, 1.387778780781445676E-14, 0.000000000000000000 ) ) ;
#4756=CARTESIAN_POINT ( 'NONE',  ( -14.19078112930533209, 29.75000000000008882, 79.50000000000000000 ) ) ;
#4760=ORIENTED_EDGE ( 'NONE', *, *, #7217, .T. ) ;
#4762=DIRECTION ( 'NONE',  ( 1.000000000000000000, 0.000000000000000000, 0.000000000000000000 ) ) ;
#4769=( NAMED_UNIT ( * ) PLANE_ANGLE_UNIT ( ) SI_UNIT ( $, .RADIAN. ) );
#4771=EDGE_CURVE ( 'NONE', #3440, #2446, #6284, .T. ) ;
#4783=ORIENTED_EDGE ( 'NONE', *, *, #19, .F. ) ;
#4784=VECTOR ( 'NONE', #3539, 1000.000000000000227 ) ;
#4792=B_SPLINE_CURVE_WITH_KNOTS ( 'NONE', 3,
 ( #4411, #4474, #3482, #1552 ),
 .UNSPECIFIED., .F., .F.,
 ( 4, 4 ),
 ( 0.0002502309401078514238, 0.0005002309401076744872 ),
 .UNSPECIFIED. ) ;
#4793=EDGE_CURVE ( 'NONE', #3205, #6749, #11243, .T. ) ;
#4796=CARTESIAN_POINT ( 'NONE',  ( -1.190781129305471087, 30.00000000000008882, 78.00000000000000000 ) ) ;
#4804=CARTESIAN_POINT ( 'NONE',  ( -5.974274778359173865, 21.21474596215567487, 79.50000000000000000 ) ) ;
#4806=EDGE_CURVE ( 'NONE', #8730, #893, #10006, .T. ) ;
#4808=VERTEX_POINT ( 'NONE', #2402 ) ;
#4823=DIRECTION ( 'NONE',  ( 1.000000000000000000, -1.040834085586083310E-14, 0.000000000000000000 ) ) ;
#4830=EDGE_CURVE ( 'NONE', #6973, #1372, #6461, .T. ) ;
#4831=CARTESIAN_POINT ( 'NONE',  ( 5.092712519748452848, 41.38333024919784719, 79.50000000000000000 ) ) ;
#4833=VERTEX_POINT ( 'NONE', #11135 ) ;
#4838=EDGE_CURVE ( 'NONE', #10836, #11371, #6215, .T. ) ;
#4841=ORIENTED_EDGE ( 'NONE', *, *, #5560, .F. ) ;
#4848=DIRECTION ( 'NONE',  ( -0.4999999999999933387, 0.8660254037844424824, 0.000000000000000000 ) ) ;
#4851=VECTOR ( 'NONE', #3094, 1000.000000000000114 ) ;
#4854=ORIENTED_EDGE ( 'NONE', *, *, #5726, .T. ) ;
#4861=VERTEX_POINT ( 'NONE', #6399 ) ;
#4864=CARTESIAN_POINT ( 'NONE',  ( 10.19254911989241386, 23.71650635094626836, 79.50000000000000000 ) ) ;
#4865=ORIENTED_EDGE ( 'NONE', *, *, #9903, .F. ) ;
#4870=LINE ( 'NONE', #8658, #7791 ) ;
#4874=AXIS2_PLACEMENT_3D ( 'NONE', #9201, #3486, #8274 ) ;
#4875=CARTESIAN_POINT ( 'NONE',  ( -0.9407811293052825707, 17.00000000000008882, 79.50000000000000000 ) ) ;
#4884=DIRECTION ( 'NONE',  ( 7.011174048739587977E-15, 1.000000000000000000, 0.000000000000000000 ) ) ;
#4887=CARTESIAN_POINT ( 'NONE',  ( 7.344472908539098732, 24.78349364905406205, 79.50000000000000000 ) ) ;
#4895=VERTEX_POINT ( 'NONE', #1726 ) ;
#4898=VERTEX_POINT ( 'NONE', #2651 ) ;
#4902=SURFACE_STYLE_USAGE ( .BOTH. , #3905 ) ;
#4904=ORIENTED_EDGE ( 'NONE', *, *, #6203, .T. ) ;
#4906=VERTEX_POINT ( 'NONE', #8378 ) ;
#4908=ORIENTED_EDGE ( 'NONE', *, *, #6422, .F. ) ;
#4910=EDGE_CURVE ( 'NONE', #2329, #2522, #2193, .T. ) ;
#4912=VECTOR ( 'NONE', #2652, 1000.000000000000000 ) ;
#4919=CARTESIAN_POINT ( 'NONE',  ( 5.092712519748611832, 18.61666975080242992, 79.50000000000000000 ) ) ;
#4922=DIRECTION ( 'NONE',  ( -0.8660254037844385966, 0.5000000000000000000, 0.000000000000000000 ) ) ;
#4938=EDGE_CURVE ( 'NONE', #4906, #4833, #11499, .T. ) ;
#4940=PLANE ( 'NONE',  #588 ) ;
#4943=CARTESIAN_POINT ( 'NONE',  ( -9.726035167149685634, 24.78349364905394125, 79.50000000000000000 ) ) ;
#4944=FACE_OUTER_BOUND ( 'NONE', #10202, .T. ) ;
#4946=ORIENTED_EDGE ( 'NONE', *, *, #996, .F. ) ;
#4950=CARTESIAN_POINT ( 'NONE',  ( -11.19078112930532853, 29.75000000000005684, 80.00000000000000000 ) ) ;
#4956=ORIENTED_EDGE ( 'NONE', *, *, #6848, .F. ) ;
#4962=FILL_AREA_STYLE_COLOUR ( '', #118 ) ;
#4965=VERTEX_POINT ( 'NONE', #2949 ) ;
#4971=CARTESIAN_POINT ( 'NONE',  ( 8.809218870694669690, 29.75000000000019540, 80.00000000000000000 ) ) ;
#4972=DIRECTION ( 'NONE',  ( 7.011174048739587977E-15, 1.000000000000000000, 0.000000000000000000 ) ) ;
#4983=ORIENTED_EDGE ( 'NONE', *, *, #2199, .T. ) ;
#5010=DIRECTION ( 'NONE',  ( 0.000000000000000000, 0.000000000000000000, -1.000000000000000000 ) ) ;
#5012=DIRECTION ( 'NONE',  ( 0.5000000000000036637, 0.8660254037844364872, 0.000000000000000000 ) ) ;
#5020=CARTESIAN_POINT ( 'NONE',  ( 11.80921887069467324, 29.75000000000018474, 79.50000000000000000 ) ) ;
#5024=DIRECTION ( 'NONE',  ( 0.8660254037844331565, -0.5000000000000095479, 0.000000000000000000 ) ) ;
#5027=( NAMED_UNIT ( * ) SI_UNIT ( $, .STERADIAN. ) SOLID_ANGLE_UNIT ( ) );
#5029=ADVANCED_FACE ( 'NONE', ( #4244 ), #11866, .F. ) ;
#5032=DIRECTION ( 'NONE',  ( 1.000000000000000000, 0.000000000000000000, 0.000000000000000000 ) ) ;
#5034=AXIS2_PLACEMENT_3D ( 'NONE', #7071, #10929, #5024 ) ;
#5046=ADVANCED_FACE ( 'NONE', ( #7176 ), #5093, .T. ) ;
#5070=PLANE ( 'NONE',  #11581 ) ;
#5078=ORIENTED_EDGE ( 'NONE', *, *, #9268, .T. ) ;
#5083=DIRECTION ( 'NONE',  ( 0.000000000000000000, 0.000000000000000000, -1.000000000000000000 ) ) ;
#5093=TOROIDAL_SURFACE ( 'NONE', #9846, 12.99999999999999822, 2.000000000000000000 ) ;
#5112=AXIS2_PLACEMENT_3D ( 'NONE', #12142, #7460, #8259 ) ;
#5118=ORIENTED_EDGE ( 'NONE', *, *, #6953, .T. ) ;
#5126=AXIS2_PLACEMENT_3D ( 'NONE', #6433, #9155, #2444 ) ;
#5127=ORIENTED_EDGE ( 'NONE', *, *, #9197, .T. ) ;
#5130=ORIENTED_EDGE ( 'NONE', *, *, #8900, .T. ) ;
#5145=ORIENTED_EDGE ( 'NONE', *, *, #9887, .T. ) ;
#5149=DIRECTION ( 'NONE',  ( -0.000000000000000000, -0.000000000000000000, 1.000000000000000000 ) ) ;
#5154=VECTOR ( 'NONE', #1990, 1000.000000000000114 ) ;
#5158=VERTEX_POINT ( 'NONE', #7488 ) ;
#5172=DIRECTION ( 'NONE',  ( -1.000000000000000000, 0.000000000000000000, -0.000000000000000000 ) ) ;
#5173=CARTESIAN_POINT ( 'NONE',  ( 5.525725221640672480, 41.13333024919784719, 80.00000000000000000 ) ) ;
#5193=CARTESIAN_POINT ( 'NONE',  ( 3.592712519748626931, 21.21474596215575659, 79.50000000000000000 ) ) ;
#5199=VECTOR ( 'NONE', #4823, 1000.000000000000000 ) ;
#5222=FACE_OUTER_BOUND ( 'NONE', #578, .T. ) ;
#5226=DIRECTION ( 'NONE',  ( 1.000000000000000000, 0.000000000000000000, -0.000000000000000000 ) ) ;
#5236=VECTOR ( 'NONE', #3264, 1000.000000000000000 ) ;
#5240=EDGE_LOOP ( 'NONE', ( #4904, #2463, #2750, #563, #369 ) ) ;
#5246=DIRECTION ( 'NONE',  ( 0.000000000000000000, 0.000000000000000000, 1.000000000000000000 ) ) ;
#5249=CARTESIAN_POINT ( 'NONE',  ( 5.091510485526559826, 18.61875173514745185, 80.00000000000000000 ) ) ;
#5254=VECTOR ( 'NONE', #10388, 1000.000000000000000 ) ;
#5256=DIRECTION ( 'NONE',  ( 0.000000000000000000, 0.000000000000000000, -1.000000000000000000 ) ) ;
#5258=EDGE_CURVE ( 'NONE', #5677, #4861, #5501, .T. ) ;
#5268=ORIENTED_EDGE ( 'NONE', *, *, #8771, .T. ) ;
#5269=FACE_OUTER_BOUND ( 'NONE', #9684, .T. ) ;
#5285=CARTESIAN_POINT ( 'NONE',  ( -14.19078112930533209, 29.75000000000008882, 80.00000000000000000 ) ) ;
#5286=CARTESIAN_POINT ( 'NONE',  ( -1.190781129305471087, 30.00000000000008882, 65.00000000000000000 ) ) ;
#5293=ORIENTED_EDGE ( 'NONE', *, *, #6485, .F. ) ;
#5297=CARTESIAN_POINT ( 'NONE',  ( 5.309218870694559556, 41.25833024919784719, 80.00000000000000000 ) ) ;
#5314=CARTESIAN_POINT ( 'NONE',  ( -0.9407811293052825707, 17.00000000000008882, 80.00000000000000000 ) ) ;
#5318=EDGE_CURVE ( 'NONE', #5385, #938, #882, .T. ) ;
#5323=DIRECTION ( 'NONE',  ( -1.000000000000000000, 0.000000000000000000, -0.000000000000000000 ) ) ;
#5330=CARTESIAN_POINT ( 'NONE',  ( -12.57411137850303540, 36.28349364905398033, 79.50000000000000000 ) ) ;
#5340=DIRECTION ( 'NONE',  ( -0.000000000000000000, -0.000000000000000000, 1.000000000000000000 ) ) ;
#5342=VECTOR ( 'NONE', #12346, 1000.000000000000114 ) ;
#5344=EDGE_CURVE ( 'NONE', #2311, #1312, #8656, .T. ) ;
#5345=ADVANCED_FACE ( 'NONE', ( #6735 ), #12324, .T. ) ;
#5350=VECTOR ( 'NONE', #8126, 1000.000000000000114 ) ;
#5352=LINE ( 'NONE', #4533, #9775 ) ;
#5354=DIRECTION ( 'NONE',  ( 0.8660254037844385966, -0.5000000000000000000, 0.000000000000000000 ) ) ;
#5356=DIRECTION ( 'NONE',  ( -1.000000000000000000, 0.000000000000000000, -0.000000000000000000 ) ) ;
#5358=ORIENTED_EDGE ( 'NONE', *, *, #3103, .F. ) ;
#5360=LINE ( 'NONE', #10962, #6164 ) ;
#5363=VERTEX_POINT ( 'NONE', #11544 ) ;
#5368=VERTEX_POINT ( 'NONE', #243 ) ;
#5375=CARTESIAN_POINT ( 'NONE',  ( 11.80921887069467324, 30.25000000000018474, 79.50000000000000000 ) ) ;
#5381=ORIENTED_EDGE ( 'NONE', *, *, #11242, .T. ) ;
#5385=VERTEX_POINT ( 'NONE', #6921 ) ;
#5406=DIRECTION ( 'NONE',  ( -0.000000000000000000, -0.000000000000000000, 1.000000000000000000 ) ) ;
#5407=AXIS2_PLACEMENT_3D ( 'NONE', #8349, #7609, #12175 ) ;
#5418=ORIENTED_EDGE ( 'NONE', *, *, #8645, .F. ) ;
#5423=LINE ( 'NONE', #619, #11032 ) ;
#5426=CARTESIAN_POINT ( 'NONE',  ( -6.407287480251453893, 38.53525403784446723, 79.50000000000000000 ) ) ;
#5427=VERTEX_POINT ( 'NONE', #2124 ) ;
#5433=CARTESIAN_POINT ( 'NONE',  ( 5.309218870694537351, 18.74166975080233044, 80.00000000000000000 ) ) ;
#5442=EDGE_CURVE ( 'NONE', #8327, #1960, #1300, .T. ) ;
#5443=ADVANCED_FACE ( 'NONE', ( #8717 ), #8257, .T. ) ;
#5445=LINE ( 'NONE', #9223, #4595 ) ;
#5460=VECTOR ( 'NONE', #1536, 1000.000000000000000 ) ;
#5462=CARTESIAN_POINT ( 'NONE',  ( 10.19254911989230727, 36.28349364905406560, 80.00000000000000000 ) ) ;
#5469=VECTOR ( 'NONE', #7442, 1000.000000000000227 ) ;
#5477=CARTESIAN_POINT ( 'NONE',  ( -0.9407811293054709756, 43.00000000000008527, 80.00000000000000000 ) ) ;
#5482=EDGE_LOOP ( 'NONE', ( #9904, #10437, #11958, #5588, #21 ) ) ;
#5489=DIRECTION ( 'NONE',  ( -0.000000000000000000, -0.000000000000000000, 1.000000000000000000 ) ) ;
#5496=VECTOR ( 'NONE', #10358, 999.9999999999998863 ) ;
#5501=LINE ( 'NONE', #764, #4256 ) ;
#5509=CARTESIAN_POINT ( 'NONE',  ( -6.407287480251391720, 21.46474596215567487, 79.50000000000000000 ) ) ;
#5514=CARTESIAN_POINT ( 'NONE',  ( -11.19078112930532853, 29.75000000000005684, 79.50000000000000000 ) ) ;
#5516=ORIENTED_EDGE ( 'NONE', *, *, #10379, .F. ) ;
#5519=ORIENTED_EDGE ( 'NONE', *, *, #7271, .T. ) ;
#5535=VERTEX_POINT ( 'NONE', #2488 ) ;
#5539=ORIENTED_EDGE ( 'NONE', *, *, #4910, .F. ) ;
#5543=DIRECTION ( 'NONE',  ( -1.000000000000000000, 0.000000000000000000, -0.000000000000000000 ) ) ;
#5559=ORIENTED_EDGE ( 'NONE', *, *, #10096, .T. ) ;
#5560=EDGE_CURVE ( 'NONE', #4906, #9416, #7102, .T. ) ;
#5570=VERTEX_POINT ( 'NONE', #428 ) ;
#5572=EDGE_CURVE ( 'NONE', #9412, #1574, #1432, .T. ) ;
#5573=DIRECTION ( 'NONE',  ( 0.8660254037844434816, 0.4999999999999913958, 0.000000000000000000 ) ) ;
#5577=ORIENTED_EDGE ( 'NONE', *, *, #513, .T. ) ;
#5578=DIRECTION ( 'NONE',  ( 0.5000000000000036637, 0.8660254037844365982, 0.000000000000000000 ) ) ;
#5580=VECTOR ( 'NONE', #2609, 1000.000000000000114 ) ;
#5587=DIRECTION ( 'NONE',  ( -1.000000000000000000, 3.469446951953611033E-15, 0.000000000000000000 ) ) ;
#5588=ORIENTED_EDGE ( 'NONE', *, *, #10184, .T. ) ;
#5591=DIRECTION ( 'NONE',  ( 0.8660254037844348218, -0.5000000000000067724, 0.000000000000000000 ) ) ;
#5602=VERTEX_POINT ( 'NONE', #12156 ) ;
#5608=ORIENTED_EDGE ( 'NONE', *, *, #3387, .T. ) ;
#5626=CARTESIAN_POINT ( 'NONE',  ( -7.474274778359196070, 18.61666975080236597, 80.00000000000000000 ) ) ;
#5635=ORIENTED_EDGE ( 'NONE', *, *, #4938, .T. ) ;
#5639=CARTESIAN_POINT ( 'NONE',  ( 8.809218870694669690, 29.75000000000019540, 79.50000000000000000 ) ) ;
#5640=CARTESIAN_POINT ( 'NONE',  ( 10.19254911989241386, 23.71650635094626836, 80.00000000000000000 ) ) ;
#5654=EDGE_CURVE ( 'NONE', #3755, #7589, #2608, .T. ) ;
#5656=CARTESIAN_POINT ( 'NONE',  ( 4.025725221640669815, 38.53525403784453118, 79.50000000000000000 ) ) ;
#5661=ORIENTED_EDGE ( 'NONE', *, *, #1611, .T. ) ;
#5662=LINE ( 'NONE', #11335, #5254 ) ;
#5671=VERTEX_POINT ( 'NONE', #4600 ) ;
#5677=VERTEX_POINT ( 'NONE', #11093 ) ;
#5689=DIRECTION ( 'NONE',  ( 1.000000000000000000, -7.011174048739587977E-15, 0.000000000000000000 ) ) ;
#5694=DIRECTION ( 'NONE',  ( -1.000000000000000000, 0.000000000000000000, -0.000000000000000000 ) ) ;
#5700=DIRECTION ( 'NONE',  ( -0.4999999999999977796, 0.8660254037844399289, 0.000000000000000000 ) ) ;
#5724=ORIENTED_EDGE ( 'NONE', *, *, #5318, .T. ) ;
#5726=EDGE_CURVE ( 'NONE', #3399, #11988, #5423, .T. ) ;
#5731=FACE_OUTER_BOUND ( 'NONE', #7366, .T. ) ;
#5741=CARTESIAN_POINT ( 'NONE',  ( 0.000000000000000000, 0.000000000000000000, 79.50000000000000000 ) ) ;
#5752=ADVANCED_FACE ( 'NONE', ( #8208 ), #12031, .T. ) ;
#5754=CARTESIAN_POINT ( 'NONE',  ( 11.80921887069467324, 29.75000000000018474, 80.00000000000000000 ) ) ;
#5764=DIRECTION ( 'NONE',  ( -0.8660254037844398178, -0.4999999999999977796, 0.000000000000000000 ) ) ;
#5793=ORIENTED_EDGE ( 'NONE', *, *, #5654, .F. ) ;
#5795=EDGE_CURVE ( 'NONE', #12197, #5535, #8762, .T. ) ;
#5796=VECTOR ( 'NONE', #900, 1000.000000000000000 ) ;
#5798=CARTESIAN_POINT ( 'NONE',  ( 10.19254911989230727, 36.28349364905406560, 79.50000000000000000 ) ) ;
#5808=ORIENTED_EDGE ( 'NONE', *, *, #1551, .T. ) ;
#5814=FACE_OUTER_BOUND ( 'NONE', #5482, .T. ) ;
#5817=DIRECTION ( 'NONE',  ( 0.4999999999999985567, 0.8660254037844394848, 0.000000000000000000 ) ) ;
#5830=( LENGTH_UNIT ( ) NAMED_UNIT ( * ) SI_UNIT ( .MILLI., .METRE. ) );
#5833=PLANE ( 'NONE',  #6088 ) ;
#5841=VECTOR ( 'NONE', #1362, 1000.000000000000000 ) ;
#5844=CARTESIAN_POINT ( 'NONE',  ( 8.809218870694669690, 30.25000000000019540, 79.50000000000000000 ) ) ;
#5847=CARTESIAN_POINT ( 'NONE',  ( -9.976035167149682081, 25.21650635094616533, 80.00000000000000000 ) ) ;
#5848=ORIENTED_EDGE ( 'NONE', *, *, #27, .F. ) ;
#5851=DIRECTION ( 'NONE',  ( -0.000000000000000000, -0.000000000000000000, 1.000000000000000000 ) ) ;
#5858=CARTESIAN_POINT ( 'NONE',  ( 7.344472908539098732, 24.78349364905406205, 80.00000000000000000 ) ) ;
#5865=CARTESIAN_POINT ( 'NONE',  ( -1.190781129305471087, 30.00000000000008882, 80.00000000000000000 ) ) ;
#5870=ORIENTED_EDGE ( 'NONE', *, *, #7210, .F. ) ;
#5872=VECTOR ( 'NONE', #3175, 1000.000000000000000 ) ;
#5874=EDGE_LOOP ( 'NONE', ( #1533, #7804, #3202, #1767, #9932 ) ) ;
#5881=DIRECTION ( 'NONE',  ( -0.8660254037844457020, -0.4999999999999877875, 0.000000000000000000 ) ) ;
#5883=EDGE_CURVE ( 'NONE', #9910, #2786, #1922, .T. ) ;
#5887=DIRECTION ( 'NONE',  ( -1.000000000000000000, 0.000000000000000000, -0.000000000000000000 ) ) ;
#5891=VECTOR ( 'NONE', #5406, 1000.000000000000000 ) ;
#5893=CARTESIAN_POINT ( 'NONE',  ( 9.942549119892305498, 36.71650635094628967, 80.00000000000000000 ) ) ;
#5897=CIRCLE ( 'NONE', #7674, 12.99999999999999822 ) ;
#5898=CARTESIAN_POINT ( 'NONE',  ( 5.524523187418778569, 18.86875173514745896, 80.00000000000000000 ) ) ;
#5899=FILL_AREA_STYLE ('',( #4962 ) ) ;
#5916=VECTOR ( 'NONE', #2077, 999.9999999999998863 ) ;
#5917=ORIENTED_EDGE ( 'NONE', *, *, #11541, .F. ) ;
#5918=ADVANCED_FACE ( 'NONE', ( #5731 ), #4722, .T. ) ;
#5922=ADVANCED_FACE ( 'NONE', ( #10519 ), #1980, .F. ) ;
#5948=EDGE_CURVE ( 'NONE', #12197, #11305, #6963, .T. ) ;
#5951=VERTEX_POINT ( 'NONE', #539 ) ;
#5958=CARTESIAN_POINT ( 'NONE',  ( -12.32411137850303184, 36.71650635094619730, 80.00000000000000000 ) ) ;
#5962=VECTOR ( 'NONE', #8456, 1000.000000000000000 ) ;
#5972=LINE ( 'NONE', #8516, #11549 ) ;
#5980=VERTEX_POINT ( 'NONE', #2226 ) ;
#5983=EDGE_LOOP ( 'NONE', ( #9014, #7002, #457, #6390 ) ) ;
#5988=DIRECTION ( 'NONE',  ( 0.5000000000000066613, 0.8660254037844347108, 0.000000000000000000 ) ) ;
#5997=EDGE_LOOP ( 'NONE', ( #4956, #7781, #10298, #1470 ) ) ;
#6000=AXIS2_PLACEMENT_3D ( 'NONE', #5375, #3506, #4246 ) ;
#6002=DIRECTION ( 'NONE',  ( 1.000000000000000000, -1.040834085586083310E-14, 0.000000000000000000 ) ) ;
#6006=CARTESIAN_POINT ( 'NONE',  ( -0.9407811293052826818, 17.00240406844413954, 80.00000000000000000 ) ) ;
#6007=AXIS2_PLACEMENT_3D ( 'NONE', #3619, #10280, #2619 ) ;
#6010=VECTOR ( 'NONE', #9318, 1000.000000000000000 ) ;
#6013=ORIENTED_EDGE ( 'NONE', *, *, #6422, .T. ) ;
#6015=CARTESIAN_POINT ( 'NONE',  ( -6.407287480251391720, 21.46474596215567487, 80.00000000000000000 ) ) ;
#6017=ORIENTED_EDGE ( 'NONE', *, *, #865, .T. ) ;
#6030=CARTESIAN_POINT ( 'NONE',  ( -1.190781129305471087, 30.00000000000008882, 78.00000000000000000 ) ) ;
#6037=CARTESIAN_POINT ( 'NONE',  ( -14.19078112930546887, 30.00000000000008882, 78.00000000000000000 ) ) ;
#6051=VECTOR ( 'NONE', #7394, 1000.000000000000000 ) ;
#6055=CARTESIAN_POINT ( 'NONE',  ( 3.592712519748626931, 21.21474596215575659, 79.50000000000000000 ) ) ;
#6058=DIRECTION ( 'NONE',  ( -0.000000000000000000, -0.000000000000000000, 1.000000000000000000 ) ) ;
#6063=LINE ( 'NONE', #7810, #2403 ) ;
#6065=DIRECTION ( 'NONE',  ( 0.8660254037844348218, -0.5000000000000067724, 0.000000000000000000 ) ) ;
#6068=VECTOR ( 'NONE', #9922, 999.9999999999998863 ) ;
#6072=ORIENTED_EDGE ( 'NONE', *, *, #7704, .F. ) ;
#6073=DIRECTION ( 'NONE',  ( -1.000000000000000000, 0.000000000000000000, 0.000000000000000000 ) ) ;
#6075=VERTEX_POINT ( 'NONE', #6277 ) ;
#6078=CARTESIAN_POINT ( 'NONE',  ( 5.092712519748611832, 18.61666975080242992, 80.00000000000000000 ) ) ;
#6088=AXIS2_PLACEMENT_3D ( 'NONE', #4831, #10499, #9615 ) ;
#6090=EDGE_CURVE ( 'NONE', #828, #12197, #10741, .T. ) ;
#6091=DIRECTION ( 'NONE',  ( -1.000000000000000000, 0.000000000000000000, 0.000000000000000000 ) ) ;
#6095=DIRECTION ( 'NONE',  ( -0.8660254037844363761, 0.5000000000000038858, 0.000000000000000000 ) ) ;
#6097=ADVANCED_FACE ( 'NONE', ( #8174 ), #9860, .F. ) ;
#6105=ORIENTED_EDGE ( 'NONE', *, *, #7536, .T. ) ;
#6108=CARTESIAN_POINT ( 'NONE',  ( 0.000000000000000000, 0.000000000000000000, 79.50000000000000000 ) ) ;
#6113=ORIENTED_EDGE ( 'NONE', *, *, #6232, .T. ) ;
#6117=LINE ( 'NONE', #1863, #8013 ) ;
#6121=ORIENTED_EDGE ( 'NONE', *, *, #8553, .T. ) ;
#6126=DIRECTION ( 'NONE',  ( -0.000000000000000000, -0.000000000000000000, 1.000000000000000000 ) ) ;
#6132=CARTESIAN_POINT ( 'NONE',  ( 10.19046713554723560, 36.28229161483199050, 80.00000000000000000 ) ) ;
#6138=APPLICATION_CONTEXT ( 'automotive_design' ) ;
#6139=CARTESIAN_POINT ( 'NONE',  ( 7.594472908538985045, 34.78349364905407270, 79.50000000000000000 ) ) ;
#6140=CARTESIAN_POINT ( 'NONE',  ( 3.592712519748626931, 21.21474596215575659, 80.00000000000000000 ) ) ;
#6145=ORIENTED_EDGE ( 'NONE', *, *, #9887, .F. ) ;
#6149=LINE ( 'NONE', #9938, #9576 ) ;
#6156=ADVANCED_FACE ( 'NONE', ( #11458 ), #11935, .T. ) ;
#6164=VECTOR ( 'NONE', #9079, 1000.000000000000000 ) ;
#6172=AXIS2_PLACEMENT_3D ( 'NONE', #7964, #10083, #8213 ) ;
#6178=LINE ( 'NONE', #2370, #22 ) ;
#6185=VERTEX_POINT ( 'NONE', #2572 ) ;
#6190=VERTEX_POINT ( 'NONE', #517 ) ;
#6192=DIRECTION ( 'NONE',  ( 1.000000000000000000, -1.387778780781445676E-14, 0.000000000000000000 ) ) ;
#6194=ADVANCED_FACE ( 'NONE', ( #3390 ), #9043, .T. ) ;
#6198=VERTEX_POINT ( 'NONE', #6132 ) ;
#6203=EDGE_CURVE ( 'NONE', #6185, #5602, #9986, .T. ) ;
#6204=VECTOR ( 'NONE', #11928, 999.9999999999998863 ) ;
#6209=AXIS2_PLACEMENT_3D ( 'NONE', #11705, #1351, #284 ) ;
#6214=CARTESIAN_POINT ( 'NONE',  ( 11.80921887069467324, 30.25000000000018474, 80.00000000000000000 ) ) ;
#6215=LINE ( 'NONE', #4459, #12262 ) ;
#6232=EDGE_CURVE ( 'NONE', #11371, #7950, #6257, .T. ) ;
#6234=ORIENTED_EDGE ( 'NONE', *, *, #10993, .T. ) ;
#6249=VECTOR ( 'NONE', #9320, 1000.000000000000227 ) ;
#6254=EDGE_CURVE ( 'NONE', #4965, #10014, #452, .T. ) ;
#6257=LINE ( 'NONE', #7126, #6068 ) ;
#6258=VECTOR ( 'NONE', #4200, 1000.000000000000000 ) ;
#6262=ORIENTED_EDGE ( 'NONE', *, *, #9673, .F. ) ;
#6269=DIRECTION ( 'NONE',  ( -0.000000000000000000, -0.000000000000000000, 1.000000000000000000 ) ) ;
#6275=CARTESIAN_POINT ( 'NONE',  ( -1.440781129305261477, 20.00000000000009592, 80.00000000000000000 ) ) ;
#6276=CARTESIAN_POINT ( 'NONE',  ( -1.190781129305471087, 43.00000000000008527, 80.00000000000000000 ) ) ;
#6277=CARTESIAN_POINT ( 'NONE',  ( -7.474274778359196070, 18.61666975080236597, 79.50000000000000000 ) ) ;
#6281=CARTESIAN_POINT ( 'NONE',  ( -1.440781129305471087, 40.00000000000008527, 79.50000000000000000 ) ) ;
#6284=CIRCLE ( 'NONE', #4480, 14.99999999999999822 ) ;
#6293=DIRECTION ( 'NONE',  ( -0.000000000000000000, -0.000000000000000000, 1.000000000000000000 ) ) ;
#6301=CARTESIAN_POINT ( 'NONE',  ( 10.19046713554732619, 23.71770838516835411, 80.00000000000000000 ) ) ;
#6302=ORIENTED_EDGE ( 'NONE', *, *, #10384, .F. ) ;
#6304=LINE ( 'NONE', #10088, #8183 ) ;
#6309=CARTESIAN_POINT ( 'NONE',  ( 5.525725221640672480, 41.13333024919784719, 79.50000000000000000 ) ) ;
#6311=ORIENTED_EDGE ( 'NONE', *, *, #1972, .T. ) ;
#6316=EDGE_CURVE ( 'NONE', #3643, #7067, #7379, .T. ) ;
#6317=EDGE_LOOP ( 'NONE', ( #1691, #11689, #9763, #650 ) ) ;
#6318=DIRECTION ( 'NONE',  ( 1.000000000000000000, 0.000000000000000000, -0.000000000000000000 ) ) ;
#6322=ORIENTED_EDGE ( 'NONE', *, *, #4621, .F. ) ;
#6330=LINE ( 'NONE', #3406, #9726 ) ;
#6347=EDGE_CURVE ( 'NONE', #9573, #6198, #3882, .T. ) ;
#6353=DIRECTION ( 'NONE',  ( 1.000000000000000000, -6.938893903907222067E-15, 0.000000000000000000 ) ) ;
#6367=ORIENTED_EDGE ( 'NONE', *, *, #7016, .T. ) ;
#6377=CIRCLE ( 'NONE', #8554, 12.99999999999999822 ) ;
#6386=VECTOR ( 'NONE', #1606, 1000.000000000000114 ) ;
#6388=ADVANCED_FACE ( 'NONE', ( #9476 ), #7557, .T. ) ;
#6390=ORIENTED_EDGE ( 'NONE', *, *, #7267, .F. ) ;
#6391=VECTOR ( 'NONE', #12191, 1000.000000000000114 ) ;
#6393=LINE ( 'NONE', #3648, #3156 ) ;
#6394=VECTOR ( 'NONE', #4884, 1000.000000000000000 ) ;
#6399=CARTESIAN_POINT ( 'NONE',  ( -1.440781129305471087, 42.99759593155604875, 80.00000000000000000 ) ) ;
#6407=VECTOR ( 'NONE', #2914, 1000.000000000000114 ) ;
#6414=CARTESIAN_POINT ( 'NONE',  ( -9.726035167149728267, 35.21650635094616888, 79.50000000000000000 ) ) ;
#6418=DIRECTION ( 'NONE',  ( 0.4999999999999878431, -0.8660254037844455910, 0.000000000000000000 ) ) ;
#6419=LINE ( 'NONE', #6539, #8535 ) ;
#6422=EDGE_CURVE ( 'NONE', #2329, #2084, #3065, .T. ) ;
#6433=CARTESIAN_POINT ( 'NONE',  ( -7.474274778359196070, 18.61666975080236597, 79.50000000000000000 ) ) ;
#6437=VECTOR ( 'NONE', #8773, 1000.000000000000000 ) ;
#6438=DIRECTION ( 'NONE',  ( -0.000000000000000000, -0.000000000000000000, 1.000000000000000000 ) ) ;
#6440=ORIENTED_EDGE ( 'NONE', *, *, #3154, .F. ) ;
#6441=CARTESIAN_POINT ( 'NONE',  ( -1.357447795992929640, 17.00000000000009592, 80.00000048127353125 ) ) ;
#6448=CARTESIAN_POINT ( 'NONE',  ( -9.726035167149728267, 35.21650635094616888, 79.50000000000000000 ) ) ;
#6460=DIRECTION ( 'NONE',  ( 0.5000000000000066613, 0.8660254037844347108, 0.000000000000000000 ) ) ;
#6461=LINE ( 'NONE', #12014, #8654 ) ;
#6466=CARTESIAN_POINT ( 'NONE',  ( -12.57411137850303540, 36.28349364905398033, 79.50000000000000000 ) ) ;
#6471=AXIS2_PLACEMENT_3D ( 'NONE', #389, #5083, #5323 ) ;
#6472=VERTEX_POINT ( 'NONE', #2187 ) ;
#6475=DIRECTION ( 'NONE',  ( 0.000000000000000000, 0.000000000000000000, -1.000000000000000000 ) ) ;
#6477=ORIENTED_EDGE ( 'NONE', *, *, #10812, .T. ) ;
#6485=EDGE_CURVE ( 'NONE', #6472, #1199, #11857, .T. ) ;
#6495=ORIENTED_EDGE ( 'NONE', *, *, #3164, .T. ) ;
#6505=ORIENTED_EDGE ( 'NONE', *, *, #8093, .F. ) ;
#6534=LINE ( 'NONE', #6414, #669 ) ;
#6539=CARTESIAN_POINT ( 'NONE',  ( -11.19078112930532498, 30.25000000000005684, 79.50000000000000000 ) ) ;
#6544=ORIENTED_EDGE ( 'NONE', *, *, #39, .T. ) ;
#6563=LINE ( 'NONE', #7559, #9227 ) ;
#6564=DIRECTION ( 'NONE',  ( -0.000000000000000000, -0.000000000000000000, 1.000000000000000000 ) ) ;
#6575=AXIS2_PLACEMENT_3D ( 'NONE', #2509, #5256, #9159 ) ;
#6578=ORIENTED_EDGE ( 'NONE', *, *, #3046, .T. ) ;
#6579=DIRECTION ( 'NONE',  ( 0.8660254037844424824, 0.4999999999999933387, 0.000000000000000000 ) ) ;
#6589=ORIENTED_EDGE ( 'NONE', *, *, #7837, .F. ) ;
#6593=LINE ( 'NONE', #3347, #2692 ) ;
#6597=DIRECTION ( 'NONE',  ( 0.000000000000000000, 0.000000000000000000, -1.000000000000000000 ) ) ;
#6598=VECTOR ( 'NONE', #6058, 1000.000000000000000 ) ;
#6600=CARTESIAN_POINT ( 'NONE',  ( -1.190781129305471087, 30.00000000000008882, 65.00000000000000000 ) ) ;
#6607=ORIENTED_EDGE ( 'NONE', *, *, #2337, .F. ) ;
#6615=ORIENTED_EDGE ( 'NONE', *, *, #608, .T. ) ;
#6624=CARTESIAN_POINT ( 'NONE',  ( 10.19254911989241386, 23.71650635094626836, 79.50000000000000000 ) ) ;
#6628=DIRECTION ( 'NONE',  ( 0.000000000000000000, 1.000000000000000000, 0.000000000000000000 ) ) ;
#6632=DIRECTION ( 'NONE',  ( 1.000000000000000000, -1.040834085586083310E-14, 0.000000000000000000 ) ) ;
#6635=EDGE_CURVE ( 'NONE', #1312, #4833, #6117, .T. ) ;
#6638=CIRCLE ( 'NONE', #1471, 12.99999999999999822 ) ;
#6639=CARTESIAN_POINT ( 'NONE',  ( -12.57202939415816267, 36.28229161483201892, 80.00000000000000000 ) ) ;
#6645=DIRECTION ( 'NONE',  ( 0.4999999999999878431, -0.8660254037844455910, 0.000000000000000000 ) ) ;
#6664=AXIS2_PLACEMENT_3D ( 'NONE', #11920, #5246, #371 ) ;
#6677=EDGE_LOOP ( 'NONE', ( #6440, #9582, #11470, #9849, #11661 ) ) ;
#6685=DIRECTION ( 'NONE',  ( -0.000000000000000000, -0.000000000000000000, 1.000000000000000000 ) ) ;
#6707=VECTOR ( 'NONE', #840, 1000.000000000000000 ) ;
#6708=CARTESIAN_POINT ( 'NONE',  ( -12.36577804515927070, 36.64433756731555292, 80.00000048127353125 ) ) ;
#6718=DIRECTION ( 'NONE',  ( -0.5000000000000005551, -0.8660254037844382635, 0.000000000000000000 ) ) ;
#6719=ORIENTED_EDGE ( 'NONE', *, *, #3352, .F. ) ;
#6725=EDGE_LOOP ( 'NONE', ( #2372, #5808, #4587, #9264, #394 ) ) ;
#6735=FACE_OUTER_BOUND ( 'NONE', #9169, .T. ) ;
#6745=CARTESIAN_POINT ( 'NONE',  ( -14.19078112930533209, 29.75000000000008882, 79.50000000000000000 ) ) ;
#6749=VERTEX_POINT ( 'NONE', #9333 ) ;
#6761=PLANE ( 'NONE',  #242 ) ;
#6762=VECTOR ( 'NONE', #6808, 1000.000000000000114 ) ;
#6766=ORIENTED_EDGE ( 'NONE', *, *, #1907, .T. ) ;
#6789=EDGE_CURVE ( 'NONE', #2446, #3440, #1654, .T. ) ;
#6790=ORIENTED_EDGE ( 'NONE', *, *, #5572, .F. ) ;
#6799=DIRECTION ( 'NONE',  ( -0.8660254037844385966, 0.5000000000000000000, 0.000000000000000000 ) ) ;
#6808=DIRECTION ( 'NONE',  ( -0.4999999999999942268, 0.8660254037844419273, 0.000000000000000000 ) ) ;
#6809=DIRECTION ( 'NONE',  ( 6.938893903907222067E-15, 1.000000000000000000, 0.000000000000000000 ) ) ;
#6814=DIRECTION ( 'NONE',  ( -0.000000000000000000, -0.000000000000000000, 1.000000000000000000 ) ) ;
#6815=DIRECTION ( 'NONE',  ( -1.000000000000000000, 0.000000000000000000, -0.000000000000000000 ) ) ;
#6817=FACE_OUTER_BOUND ( 'NONE', #2204, .T. ) ;
#6821=( NAMED_UNIT ( * ) SI_UNIT ( $, .STERADIAN. ) SOLID_ANGLE_UNIT ( ) );
#6825=VECTOR ( 'NONE', #1965, 1000.000000000000114 ) ;
#6834=ORIENTED_EDGE ( 'NONE', *, *, #7572, .F. ) ;
#6837=EDGE_CURVE ( 'NONE', #632, #4906, #237, .T. ) ;
#6838=LINE ( 'NONE', #4971, #2254 ) ;
#6848=EDGE_CURVE ( 'NONE', #5951, #434, #47, .T. ) ;
#6853=DIRECTION ( 'NONE',  ( 0.8660254037844331565, -0.5000000000000095479, 0.000000000000000000 ) ) ;
#6863=EDGE_CURVE ( 'NONE', #6075, #10718, #11536, .T. ) ;
#6872=VECTOR ( 'NONE', #6192, 1000.000000000000000 ) ;
#6874=CARTESIAN_POINT ( 'NONE',  ( 9.942549119892305498, 36.71650635094628967, 79.50000000000000000 ) ) ;
#6878=LINE ( 'NONE', #10793, #11773 ) ;
#6883=ORIENTED_EDGE ( 'NONE', *, *, #3454, .F. ) ;
#6892=VECTOR ( 'NONE', #3835, 1000.000000000000000 ) ;
#6896=DIRECTION ( 'NONE',  ( 0.5000000000000066613, 0.8660254037844347108, 0.000000000000000000 ) ) ;
#6909=CARTESIAN_POINT ( 'NONE',  ( 10.06754911989233392, 36.50000000000012079, 80.00000000000000000 ) ) ;
#6913=VERTEX_POINT ( 'NONE', #10016 ) ;
#6920=EDGE_CURVE ( 'NONE', #10198, #1420, #11964, .T. ) ;
#6921=CARTESIAN_POINT ( 'NONE',  ( 5.525725221640672480, 41.13333024919784719, 80.00000000000000000 ) ) ;
#6923=EDGE_LOOP ( 'NONE', ( #3320, #2302, #4120, #4015 ) ) ;
#6926=ORIENTED_EDGE ( 'NONE', *, *, #3164, .F. ) ;
#6940=DIRECTION ( 'NONE',  ( 0.5000000000000066613, 0.8660254037844347108, 0.000000000000000000 ) ) ;
#6942=EDGE_CURVE ( 'NONE', #2274, #12042, #546, .T. ) ;
#6947=DIRECTION ( 'NONE',  ( -0.000000000000000000, -0.000000000000000000, 1.000000000000000000 ) ) ;
#6952=CARTESIAN_POINT ( 'NONE',  ( -7.907287480251413925, 18.86666975080236597, 80.00000000000000000 ) ) ;
#6953=EDGE_CURVE ( 'NONE', #11346, #4808, #486, .T. ) ;
#6963=LINE ( 'NONE', #8885, #2672 ) ;
#6966=ORIENTED_EDGE ( 'NONE', *, *, #10414, .F. ) ;
#6972=DIRECTION ( 'NONE',  ( -0.000000000000000000, -0.000000000000000000, 1.000000000000000000 ) ) ;
#6973=VERTEX_POINT ( 'NONE', #9827 ) ;
#6974=CARTESIAN_POINT ( 'NONE',  ( -0.9407811293052825707, 17.00000000000008882, 79.50000000000000000 ) ) ;
#6983=ADVANCED_FACE ( 'NONE', ( #2295 ), #7220, .T. ) ;
#6996=ORIENTED_EDGE ( 'NONE', *, *, #2689, .T. ) ;
#7002=ORIENTED_EDGE ( 'NONE', *, *, #12198, .F. ) ;
#7010=ORIENTED_EDGE ( 'NONE', *, *, #681, .F. ) ;
#7016=EDGE_CURVE ( 'NONE', #11371, #10583, #358, .T. ) ;
#7030=CIRCLE ( 'NONE', #3852, 12.99999999999999822 ) ;
#7031=DIRECTION ( 'NONE',  ( -0.4999999999999985012, -0.8660254037844394848, 0.000000000000000000 ) ) ;
#7032=ORIENTED_EDGE ( 'NONE', *, *, #10384, .T. ) ;
#7056=AXIS2_PLACEMENT_3D ( 'NONE', #8515, #12337, #9509 ) ;
#7060=CARTESIAN_POINT ( 'NONE',  ( -1.440781129305471087, 43.00000000000008527, 79.50000000000000000 ) ) ;
#7067=VERTEX_POINT ( 'NONE', #8268 ) ;
#7070=ORIENTED_EDGE ( 'NONE', *, *, #9714, .F. ) ;
#7071=CARTESIAN_POINT ( 'NONE',  ( -12.57411137850303540, 36.28349364905398033, 79.50000000000000000 ) ) ;
#7081=AXIS2_PLACEMENT_3D ( 'NONE', #8729, #191, #3821 ) ;
#7082=CARTESIAN_POINT ( 'NONE',  ( 10.10921578655968922, 36.42783121635022781, 80.00000000000000000 ) ) ;
#7083=EDGE_CURVE ( 'NONE', #3881, #5427, #6534, .T. ) ;
#7086=CARTESIAN_POINT ( 'NONE',  ( -7.907287480251413925, 18.86666975080236597, 79.50000000000000000 ) ) ;
#7102=LINE ( 'NONE', #11721, #11444 ) ;
#7124=VECTOR ( 'NONE', #7357, 1000.000000000000000 ) ;
#7126=CARTESIAN_POINT ( 'NONE',  ( 5.092712519748452848, 41.38333024919784719, 80.00000000000000000 ) ) ;
#7131=CARTESIAN_POINT ( 'NONE',  ( 5.164881303379191380, 18.65833641745863147, 80.00000048127353125 ) ) ;
#7141=EDGE_CURVE ( 'NONE', #4861, #7589, #6638, .T. ) ;
#7143=DIRECTION ( 'NONE',  ( -0.000000000000000000, -0.000000000000000000, -1.000000000000000000 ) ) ;
#7145=DIRECTION ( 'NONE',  ( -0.000000000000000000, -0.000000000000000000, 1.000000000000000000 ) ) ;
#7153=ADVANCED_FACE ( 'NONE', ( #2544 ), #862, .T. ) ;
#7154=EDGE_CURVE ( 'NONE', #11256, #5951, #5662, .T. ) ;
#7168=AXIS2_PLACEMENT_3D ( 'NONE', #3077, #6065, #6940 ) ;
#7173=DIRECTION ( 'NONE',  ( -0.8660254037844363761, 0.5000000000000038858, 0.000000000000000000 ) ) ;
#7176=FACE_OUTER_BOUND ( 'NONE', #11925, .T. ) ;
#7186=VECTOR ( 'NONE', #8973, 1000.000000000000000 ) ;
#7189=ORIENTED_EDGE ( 'NONE', *, *, #9406, .T. ) ;
#7196=DIRECTION ( 'NONE',  ( 0.8660254037844434816, 0.4999999999999913958, 0.000000000000000000 ) ) ;
#7197=VECTOR ( 'NONE', #5988, 1000.000000000000114 ) ;
#7203=DIRECTION ( 'NONE',  ( -1.000000000000000000, 3.469446951953611033E-15, 0.000000000000000000 ) ) ;
#7207=LINE ( 'NONE', #9310, #8950 ) ;
#7210=EDGE_CURVE ( 'NONE', #8730, #11587, #985, .T. ) ;
#7214=EDGE_CURVE ( 'NONE', #2747, #11089, #1043, .T. ) ;
#7217=EDGE_CURVE ( 'NONE', #9910, #3039, #7767, .T. ) ;
#7220=PLANE ( 'NONE',  #12216 ) ;
#7225=VECTOR ( 'NONE', #7031, 1000.000000000000114 ) ;
#7241=EDGE_CURVE ( 'NONE', #11844, #11089, #6838, .T. ) ;
#7244=DIRECTION ( 'NONE',  ( -1.000000000000000000, 1.387778780781445676E-14, 0.000000000000000000 ) ) ;
#7247=ORIENTED_EDGE ( 'NONE', *, *, #7083, .T. ) ;
#7253=DIRECTION ( 'NONE',  ( 0.4999999999999977796, -0.8660254037844399289, 0.000000000000000000 ) ) ;
#7255=ORIENTED_EDGE ( 'NONE', *, *, #11133, .T. ) ;
#7259=ORIENTED_EDGE ( 'NONE', *, *, #10274, .F. ) ;
#7265=VERTEX_POINT ( 'NONE', #96 ) ;
#7267=EDGE_CURVE ( 'NONE', #828, #5368, #10450, .T. ) ;
#7269=CARTESIAN_POINT ( 'NONE',  ( 9.942549119892305498, 36.71650635094628967, 80.00000000000000000 ) ) ;
#7270=CARTESIAN_POINT ( 'NONE',  ( 10.02588245322500882, 23.42783121635017451, 80.00000000000000000 ) ) ;
#7271=EDGE_CURVE ( 'NONE', #6973, #301, #1917, .T. ) ;
#7273=LINE ( 'NONE', #10062, #10381 ) ;
#7276=PLANE ( 'NONE',  #5112 ) ;
#7282=VECTOR ( 'NONE', #6632, 1000.000000000000000 ) ;
#7305=CARTESIAN_POINT ( 'NONE',  ( -9.976035167149682081, 25.21650635094616533, 79.50000000000000000 ) ) ;
#7310=LINE ( 'NONE', #5193, #7186 ) ;
#7313=DIRECTION ( 'NONE',  ( 0.8660254037844377084, -0.5000000000000015543, 0.000000000000000000 ) ) ;
#7331=DIRECTION ( 'NONE',  ( -0.8660254037844398178, -0.4999999999999977796, 0.000000000000000000 ) ) ;
#7355=LINE ( 'NONE', #2611, #4589 ) ;
#7357=DIRECTION ( 'NONE',  ( 7.011174048739587977E-15, 1.000000000000000000, 0.000000000000000000 ) ) ;
#7359=DIRECTION ( 'NONE',  ( -0.8660254037844363761, 0.5000000000000038858, 0.000000000000000000 ) ) ;
#7364=CARTESIAN_POINT ( 'NONE',  ( -1.440781129305471087, 43.00000000000008527, 79.50000000000000000 ) ) ;
#7366=EDGE_LOOP ( 'NONE', ( #220, #10233, #6766, #2336, #821 ) ) ;
#7373=ADVANCED_FACE ( 'NONE', ( #4151 ), #7885, .T. ) ;
#7378=CARTESIAN_POINT ( 'NONE',  ( 0.000000000000000000, 0.000000000000000000, 79.50000000000000000 ) ) ;
#7379=LINE ( 'NONE', #2878, #8840 ) ;
#7381=CARTESIAN_POINT ( 'NONE',  ( 5.092712519748452848, 41.38333024919784719, 79.50000000000000000 ) ) ;
#7383=EDGE_LOOP ( 'NONE', ( #9289, #11216, #11732, #518 ) ) ;
#7384=PLANE ( 'NONE',  #9795 ) ;
#7393=EDGE_CURVE ( 'NONE', #5602, #872, #7030, .T. ) ;
#7394=DIRECTION ( 'NONE',  ( 7.011174048739587977E-15, 1.000000000000000000, 0.000000000000000000 ) ) ;
#7395=CARTESIAN_POINT ( 'NONE',  ( -9.976035167149682081, 25.21650635094616533, 79.50000000000000000 ) ) ;
#7406=DIRECTION ( 'NONE',  ( 3.469446951953611033E-15, 1.000000000000000000, 0.000000000000000000 ) ) ;
#7408=VECTOR ( 'NONE', #10407, 1000.000000000000000 ) ;
#7417=PLANE ( 'NONE',  #11742 ) ;
#7419=DIRECTION ( 'NONE',  ( -1.000000000000000000, 1.387778780781445676E-14, 0.000000000000000000 ) ) ;
#7421=EDGE_CURVE ( 'NONE', #5427, #11988, #468, .T. ) ;
#7429=ORIENTED_EDGE ( 'NONE', *, *, #701, .T. ) ;
#7433=PLANE ( 'NONE',  #2808 ) ;
#7436=VECTOR ( 'NONE', #6972, 1000.000000000000000 ) ;
#7442=DIRECTION ( 'NONE',  ( -0.8660254037844403729, -0.4999999999999970024, 0.000000000000000000 ) ) ;
#7445=VERTEX_POINT ( 'NONE', #407 ) ;
#7446=CARTESIAN_POINT ( 'NONE',  ( -6.407287480251453893, 38.53525403784446723, 80.00000000000000000 ) ) ;
#7452=VECTOR ( 'NONE', #6947, 1000.000000000000000 ) ;
#7454=CARTESIAN_POINT ( 'NONE',  ( -14.18837706086142525, 29.75000000000008882, 80.00000000000000000 ) ) ;
#7459=CARTESIAN_POINT ( 'NONE',  ( -14.19078112930533031, 30.08333333333487403, 80.00000000000000000 ) ) ;
#7460=DIRECTION ( 'NONE',  ( 0.000000000000000000, 1.000000000000000000, 0.000000000000000000 ) ) ;
#7461=PLANE ( 'NONE',  #2828 ) ;
#7470=CARTESIAN_POINT ( 'NONE',  ( -12.57411137850303540, 36.28349364905398033, 80.00000000000000000 ) ) ;
#7471=ORIENTED_EDGE ( 'NONE', *, *, #8287, .T. ) ;
#7473=CARTESIAN_POINT ( 'NONE',  ( 0.000000000000000000, 0.000000000000000000, 79.50000000000000000 ) ) ;
#7476=FACE_OUTER_BOUND ( 'NONE', #3162, .T. ) ;
#7481=ORIENTED_EDGE ( 'NONE', *, *, #8924, .T. ) ;
#7486=EDGE_LOOP ( 'NONE', ( #1, #2942, #12266, #9135, #4306 ) ) ;
#7488=CARTESIAN_POINT ( 'NONE',  ( 10.19254911989230727, 36.28349364905406560, 79.50000000000000000 ) ) ;
#7496=CARTESIAN_POINT ( 'NONE',  ( -0.9407811293054709756, 40.00000000000008527, 79.50000000000000000 ) ) ;
#7508=VECTOR ( 'NONE', #6628, 1000.000000000000000 ) ;
#7509=ORIENTED_EDGE ( 'NONE', *, *, #3844, .T. ) ;
#7514=CARTESIAN_POINT ( 'NONE',  ( 4.025725221640669815, 38.53525403784453118, 80.00000000000000000 ) ) ;
#7517=CARTESIAN_POINT ( 'NONE',  ( -6.407287480251391720, 21.46474596215567487, 79.50000000000000000 ) ) ;
#7521=EDGE_CURVE ( 'NONE', #3440, #1199, #11074, .T. ) ;
#7522=UNCERTAINTY_MEASURE_WITH_UNIT (LENGTH_MEASURE( 1.000000000000000082E-05 ), #5830, 'distance_accuracy_value', 'NONE');
#7527=DIRECTION ( 'NONE',  ( 0.000000000000000000, 0.000000000000000000, -1.000000000000000000 ) ) ;
#7534=DIRECTION ( 'NONE',  ( -0.8660254037844403729, -0.4999999999999970579, 0.000000000000000000 ) ) ;
#7535=VECTOR ( 'NONE', #20, 1000.000000000000114 ) ;
#7536=EDGE_CURVE ( 'NONE', #2084, #11256, #4525, .T. ) ;
#7540=CARTESIAN_POINT ( 'NONE',  ( 5.092712519748611832, 18.61666975080242992, 80.00000000000000000 ) ) ;
#7545=DIRECTION ( 'NONE',  ( -0.5000000000000006661, -0.8660254037844383745, 0.000000000000000000 ) ) ;
#7546=CARTESIAN_POINT ( 'NONE',  ( 11.80681480225048396, 30.25000000000018474, 80.00000000000000000 ) ) ;
#7547=DIRECTION ( 'NONE',  ( 1.387778780781445676E-14, 1.000000000000000000, 0.000000000000000000 ) ) ;
#7550=VERTEX_POINT ( 'NONE', #7514 ) ;
#7554=VECTOR ( 'NONE', #10665, 1000.000000000000000 ) ;
#7556=FACE_OUTER_BOUND ( 'NONE', #8051, .T. ) ;
#7557=PLANE ( 'NONE',  #10443 ) ;
#7559=CARTESIAN_POINT ( 'NONE',  ( 5.092712519748452848, 41.38333024919784719, 80.00000000000000000 ) ) ;
#7572=EDGE_CURVE ( 'NONE', #1420, #11972, #4337, .T. ) ;
#7574=ORIENTED_EDGE ( 'NONE', *, *, #8369, .T. ) ;
#7577=LINE ( 'NONE', #5656, #4415 ) ;
#7582=FACE_OUTER_BOUND ( 'NONE', #10521, .T. ) ;
#7586=CARTESIAN_POINT ( 'NONE',  ( -12.32411137850302119, 23.28349364905396612, 79.50000000000000000 ) ) ;
#7589=VERTEX_POINT ( 'NONE', #2712 ) ;
#7598=ORIENTED_EDGE ( 'NONE', *, *, #9659, .T. ) ;
#7603=FACE_OUTER_BOUND ( 'NONE', #10890, .T. ) ;
#7604=ORIENTED_EDGE ( 'NONE', *, *, #9673, .T. ) ;
#7605=EDGE_CURVE ( 'NONE', #11491, #10191, #12261, .T. ) ;
#7609=DIRECTION ( 'NONE',  ( -0.8660254037844365982, 0.5000000000000036637, 0.000000000000000000 ) ) ;
#7629=VERTEX_POINT ( 'NONE', #23 ) ;
#7630=SURFACE_STYLE_FILL_AREA ( #8490 ) ;
#7636=DIRECTION ( 'NONE',  ( 1.000000000000000000, 0.000000000000000000, 0.000000000000000000 ) ) ;
#7647=DIRECTION ( 'NONE',  ( 0.000000000000000000, 1.000000000000000000, 0.000000000000000000 ) ) ;
#7657=AXIS2_PLACEMENT_3D ( 'NONE', #7473, #8269, #5543 ) ;
#7659=LINE ( 'NONE', #7540, #5154 ) ;
#7670=ORIENTED_EDGE ( 'NONE', *, *, #832, .T. ) ;
#7674=AXIS2_PLACEMENT_3D ( 'NONE', #12188, #3635, #2823 ) ;
#7678=CLOSED_SHELL ( 'NONE', ( #7373, #5046, #5443, #3513, #6388, #5922, #2596, #10693, #9109, #8609, #2550, #3804, #6194, #11655, #11853, #10430, #7905, #8981, #3814, #10658, #5029, #9161, #11146, #476, #717, #4450, #3500, #6983, #8448, #5345, #1835, #3731, #9949, #12118, #5752, #7985, #10490, #2569, #12326, #7153, #10340, #1553, #8220, #8822, #1433, #4329, #377, #3132, #1051, #1639, #6097, #295, #10722, #1871, #6156, #11189, #8629, #9408, #11378, #10196, #4195, #10154, #7699, #5918, #4061, #11570 ) ) ;
#7687=DIRECTION ( 'NONE',  ( 0.000000000000000000, 0.000000000000000000, 1.000000000000000000 ) ) ;
#7691=EDGE_CURVE ( 'NONE', #1251, #632, #7758, .T. ) ;
#7692=FILL_AREA_STYLE_COLOUR ( '', #11117 ) ;
#7699=ADVANCED_FACE ( 'NONE', ( #3902 ), #6761, .T. ) ;
#7701=( LENGTH_UNIT ( ) NAMED_UNIT ( * ) SI_UNIT ( .MILLI., .METRE. ) );
#7704=EDGE_CURVE ( 'NONE', #5602, #1941, #9679, .T. ) ;
#7721=EDGE_LOOP ( 'NONE', ( #11046, #8727, #2849, #372, #11284, #139, #168, #11735, #2296, #9907, #3830, #919, #11580, #1101, #1161, #5917, #3239, #7189, #3109, #3059, #7908, #11921, #1012, #2757, #5559, #12110, #10782, #9292, #7574, #2450, #8574, #11602, #5130 ) ) ;
#7724=ORIENTED_EDGE ( 'NONE', *, *, #5795, .F. ) ;
#7727=CARTESIAN_POINT ( 'NONE',  ( -1.440781129305282571, 17.00240406844413243, 80.00000000000000000 ) ) ;
#7730=CARTESIAN_POINT ( 'NONE',  ( 11.80921887069467324, 29.91666666666539953, 80.00000000000000000 ) ) ;
#7732=CARTESIAN_POINT ( 'NONE',  ( 3.592712519748450628, 38.78525403784453118, 79.50000000000000000 ) ) ;
#7745=DIRECTION ( 'NONE',  ( -0.000000000000000000, -0.000000000000000000, 1.000000000000000000 ) ) ;
#7758=LINE ( 'NONE', #10501, #6825 ) ;
#7760=CARTESIAN_POINT ( 'NONE',  ( -1.190781129305471087, 30.00000000000008882, 80.00000000000000000 ) ) ;
#7763=EDGE_CURVE ( 'NONE', #5980, #11423, #1341, .T. ) ;
#7764=ORIENTED_EDGE ( 'NONE', *, *, #8287, .F. ) ;
#7765=EDGE_CURVE ( 'NONE', #6973, #6185, #4320, .T. ) ;
#7767=LINE ( 'NONE', #1975, #10015 ) ;
#7774=VECTOR ( 'NONE', #1762, 1000.000000000000000 ) ;
#7776=ORIENTED_EDGE ( 'NONE', *, *, #3705, .F. ) ;
#7781=ORIENTED_EDGE ( 'NONE', *, *, #7154, .F. ) ;
#7782=CARTESIAN_POINT ( 'NONE',  ( 5.525725221640833240, 18.86666975080242992, 80.00000000000000000 ) ) ;
#7787=ORIENTED_EDGE ( 'NONE', *, *, #11055, .T. ) ;
#7791=VECTOR ( 'NONE', #2996, 1000.000000000000114 ) ;
#7795=DIRECTION ( 'NONE',  ( 7.011174048739587977E-15, 1.000000000000000000, 0.000000000000000000 ) ) ;
#7804=ORIENTED_EDGE ( 'NONE', *, *, #7605, .T. ) ;
#7810=CARTESIAN_POINT ( 'NONE',  ( -0.9407811293052614765, 20.00000000000009237, 79.50000000000000000 ) ) ;
#7821=CARTESIAN_POINT ( 'NONE',  ( -1.440781129305471087, 43.00000000000008527, 79.50000000000000000 ) ) ;
#7823=DIRECTION ( 'NONE',  ( 0.000000000000000000, 0.000000000000000000, 1.000000000000000000 ) ) ;
#7836=CARTESIAN_POINT ( 'NONE',  ( 5.525725221640672480, 41.13333024919784719, 79.50000000000000000 ) ) ;
#7837=EDGE_CURVE ( 'NONE', #8588, #10191, #11822, .T. ) ;
#7840=LINE ( 'NONE', #533, #5350 ) ;
#7845=ORIENTED_EDGE ( 'NONE', *, *, #2199, .F. ) ;
#7859=DIRECTION ( 'NONE',  ( -0.8660254037844399289, -0.4999999999999977796, 0.000000000000000000 ) ) ;
#7864=CARTESIAN_POINT ( 'NONE',  ( 5.525725221640672480, 41.13333024919784719, 79.50000000000000000 ) ) ;
#7867=CARTESIAN_POINT ( 'NONE',  ( -7.618612345655469298, 41.29999691586513677, 80.00000000000000000 ) ) ;
#7872=PRODUCT_DEFINITION_SHAPE ( 'NONE', 'NONE',  #3674 ) ;
#7885=CYLINDRICAL_SURFACE ( 'NONE', #3061, 15.00000000000000000 ) ;
#7887=DIRECTION ( 'NONE',  ( 0.8660254037844331565, -0.5000000000000095479, 0.000000000000000000 ) ) ;
#7905=ADVANCED_FACE ( 'NONE', ( #5269 ), #10869, .F. ) ;
#7906=ORIENTED_EDGE ( 'NONE', *, *, #200, .T. ) ;
#7908=ORIENTED_EDGE ( 'NONE', *, *, #3662, .F. ) ;
#7911=EDGE_LOOP ( 'NONE', ( #4243, #815, #8875, #5539, #15 ) ) ;
#7915=ORIENTED_EDGE ( 'NONE', *, *, #6347, .F. ) ;
#7916=EDGE_CURVE ( 'NONE', #1468, #3039, #1522, .T. ) ;
#7935=EDGE_LOOP ( 'NONE', ( #3694, #5516, #4296, #296, #7776 ) ) ;
#7939=CIRCLE ( 'NONE', #9532, 2.000000000000001776 ) ;
#7942=CARTESIAN_POINT ( 'NONE',  ( -9.726035167149728267, 35.21650635094616888, 80.00000000000000000 ) ) ;
#7950=VERTEX_POINT ( 'NONE', #10051 ) ;
#7951=CARTESIAN_POINT ( 'NONE',  ( 10.19254911989230727, 36.28349364905406560, 79.50000000000000000 ) ) ;
#7955=VECTOR ( 'NONE', #11530, 1000.000000000000114 ) ;
#7956=CARTESIAN_POINT ( 'NONE',  ( 5.092712519748452848, 41.38333024919784719, 80.00000000000000000 ) ) ;
#7964=CARTESIAN_POINT ( 'NONE',  ( -7.474274778359198734, 41.38333024919781167, 79.50000000000000000 ) ) ;
#7974=LINE ( 'NONE', #9786, #10470 ) ;
#7985=ADVANCED_FACE ( 'NONE', ( #7603 ), #7384, .F. ) ;
#7990=VERTEX_POINT ( 'NONE', #9106 ) ;
#7991=LINE ( 'NONE', #6015, #12236 ) ;
#8001=ORIENTED_EDGE ( 'NONE', *, *, #5883, .F. ) ;
#8005=PLANE ( 'NONE',  #12192 ) ;
#8013=VECTOR ( 'NONE', #7359, 1000.000000000000114 ) ;
#8015=FACE_OUTER_BOUND ( 'NONE', #9875, .T. ) ;
#8026=ORIENTED_EDGE ( 'NONE', *, *, #4830, .T. ) ;
#8028=VECTOR ( 'NONE', #8373, 1000.000000000000114 ) ;
#8029=AXIS2_PLACEMENT_3D ( 'NONE', #1571, #378, #1509 ) ;
#8039=CARTESIAN_POINT ( 'NONE',  ( -1.190781129305471087, 30.00000000000008882, 78.00000000000000000 ) ) ;
#8050=CARTESIAN_POINT ( 'NONE',  ( -1.440781129305261477, 20.00000000000009592, 79.50000000000000000 ) ) ;
#8051=EDGE_LOOP ( 'NONE', ( #1124, #7509, #4248, #8453, #10987 ) ) ;
#8052=PLANE ( 'NONE',  #78 ) ;
#8063=ORIENTED_EDGE ( 'NONE', *, *, #10812, .F. ) ;
#8066=FACE_OUTER_BOUND ( 'NONE', #5997, .T. ) ;
#8071=CARTESIAN_POINT ( 'NONE',  ( 8.809218870694669690, 29.75000000000019540, 79.50000000000000000 ) ) ;
#8080=MECHANICAL_DESIGN_GEOMETRIC_PRESENTATION_REPRESENTATION('',(#9473),#10876);
#8093=EDGE_CURVE ( 'NONE', #1574, #3208, #4110, .T. ) ;
#8097=PLANE ( 'NONE',  #11385 ) ;
#8103=ORIENTED_EDGE ( 'NONE', *, *, #7421, .T. ) ;
#8108=VECTOR ( 'NONE', #6853, 1000.000000000000114 ) ;
#8111=ORIENTED_EDGE ( 'NONE', *, *, #11055, .F. ) ;
#8112=FACE_OUTER_BOUND ( 'NONE', #6677, .T. ) ;
#8116=CARTESIAN_POINT ( 'NONE',  ( -12.32411137850302119, 23.28349364905396612, 79.50000000000000000 ) ) ;
#8118=LINE ( 'NONE', #275, #11084 ) ;
#8124=UNCERTAINTY_MEASURE_WITH_UNIT (LENGTH_MEASURE( 1.000000000000000082E-05 ), #7701, 'distance_accuracy_value', 'NONE');
#8126=DIRECTION ( 'NONE',  ( -0.4999999999999985012, 0.8660254037844394848, 0.000000000000000000 ) ) ;
#8132=DIRECTION ( 'NONE',  ( 7.011174048739587977E-15, 1.000000000000000000, 0.000000000000000000 ) ) ;
#8137=PLANE ( 'NONE',  #3196 ) ;
#8143=ORIENTED_EDGE ( 'NONE', *, *, #11334, .T. ) ;
#8147=AXIS2_PLACEMENT_3D ( 'NONE', #9450, #4602, #1678 ) ;
#8152=CIRCLE ( 'NONE', #10948, 14.99999999999999822 ) ;
#8161=VECTOR ( 'NONE', #3825, 1000.000000000000000 ) ;
#8162=CARTESIAN_POINT ( 'NONE',  ( -12.32411137850303184, 36.71650635094619730, 79.50000000000000000 ) ) ;
#8173=ORIENTED_EDGE ( 'NONE', *, *, #11797, .F. ) ;
#8174=FACE_OUTER_BOUND ( 'NONE', #9656, .T. ) ;
#8183=VECTOR ( 'NONE', #1566, 1000.000000000000114 ) ;
#8185=B_SPLINE_CURVE_WITH_KNOTS ( 'NONE', 3,
 ( #5297, #11908, #2420, #5173 ),
 .UNSPECIFIED., .F., .F.,
 ( 4, 4 ),
 ( 0.0002502309401076743193, 0.0005002309401076760051 ),
 .UNSPECIFIED. ) ;
#8187=LINE ( 'NONE', #1721, #10026 ) ;
#8208=FACE_OUTER_BOUND ( 'NONE', #6317, .T. ) ;
#8209=LINE ( 'NONE', #10269, #5580 ) ;
#8213=DIRECTION ( 'NONE',  ( 0.4999999999999877875, -0.8660254037844457020, 0.000000000000000000 ) ) ;
#8220=ADVANCED_FACE ( 'NONE', ( #11480 ), #1994, .T. ) ;
#8226=LINE ( 'NONE', #6309, #6204 ) ;
#8230=PLANE ( 'NONE',  #6575 ) ;
#8232=EDGE_LOOP ( 'NONE', ( #687, #756, #5127, #11163 ) ) ;
#8236=VERTEX_POINT ( 'NONE', #7727 ) ;
#8239=DIRECTION ( 'NONE',  ( 0.8660254037844385966, -0.5000000000000000000, 0.000000000000000000 ) ) ;
#8248=ORIENTED_EDGE ( 'NONE', *, *, #8808, .T. ) ;
#8257=TOROIDAL_SURFACE ( 'NONE', #4483, 12.99999999999999822, 2.000000000000000000 ) ;
#8259=DIRECTION ( 'NONE',  ( 0.000000000000000000, -0.000000000000000000, 1.000000000000000000 ) ) ;
#8268=CARTESIAN_POINT ( 'NONE',  ( -12.57202939415815202, 23.71770838516814450, 80.00000000000000000 ) ) ;
#8269=DIRECTION ( 'NONE',  ( 0.000000000000000000, 0.000000000000000000, -1.000000000000000000 ) ) ;
#8271=ORIENTED_EDGE ( 'NONE', *, *, #713, .F. ) ;
#8274=DIRECTION ( 'NONE',  ( -0.4999999999999985567, 0.8660254037844394848, 0.000000000000000000 ) ) ;
#8276=CARTESIAN_POINT ( 'NONE',  ( -7.907287480251413925, 18.86666975080236597, 79.50000000000000000 ) ) ;
#8286=ORIENTED_EDGE ( 'NONE', *, *, #11916, .F. ) ;
#8287=EDGE_CURVE ( 'NONE', #10583, #5385, #8185, .T. ) ;
#8304=ORIENTED_EDGE ( 'NONE', *, *, #9714, .T. ) ;
#8307=LINE ( 'NONE', #9482, #5796 ) ;
#8309=ORIENTED_EDGE ( 'NONE', *, *, #6837, .T. ) ;
#8327=VERTEX_POINT ( 'NONE', #10322 ) ;
#8341=ORIENTED_EDGE ( 'NONE', *, *, #11085, .F. ) ;
#8345=EDGE_LOOP ( 'NONE', ( #6072, #4123, #5577, #2711, #8864, #3274, #11231, #11727, #1867, #11599, #6996, #8304, #1179, #11251, #3120, #6578, #11615, #9961, #11384, #4673, #4865, #8744, #9719, #611, #3124, #7787, #17, #12099, #8686, #100, #6234, #11979, #162, #1625, #7604, #1699, #10784, #8143, #156, #8103, #1487, #11998, #10635, #8993, #6883, #10345, #67, #8420 ) ) ;
#8349=CARTESIAN_POINT ( 'NONE',  ( -9.726035167149728267, 35.21650635094616888, 79.50000000000000000 ) ) ;
#8350=ORIENTED_EDGE ( 'NONE', *, *, #2614, .T. ) ;
#8365=CARTESIAN_POINT ( 'NONE',  ( 5.525725221640833240, 18.86666975080242992, 79.50000000000000000 ) ) ;
#8369=EDGE_CURVE ( 'NONE', #10487, #3643, #4036, .T. ) ;
#8373=DIRECTION ( 'NONE',  ( 0.5000000000000066613, 0.8660254037844347108, 0.000000000000000000 ) ) ;
#8378=CARTESIAN_POINT ( 'NONE',  ( 7.344472908539098732, 24.78349364905406205, 79.50000000000000000 ) ) ;
#8382=LINE ( 'NONE', #4648, #10382 ) ;
#8384=CARTESIAN_POINT ( 'NONE',  ( 10.19254911989241386, 23.71650635094626836, 80.00000000000000000 ) ) ;
#8401=ORIENTED_EDGE ( 'NONE', *, *, #19, .T. ) ;
#8405=VERTEX_POINT ( 'NONE', #3724 ) ;
#8411=CARTESIAN_POINT ( 'NONE',  ( 7.594472908539098732, 25.21650635094628257, 79.50000000000000000 ) ) ;
#8420=ORIENTED_EDGE ( 'NONE', *, *, #8449, .T. ) ;
#8432=VECTOR ( 'NONE', #6073, 1000.000000000000000 ) ;
#8437=CARTESIAN_POINT ( 'NONE',  ( -7.474274778359196070, 18.61666975080236597, 79.50000000000000000 ) ) ;
#8448=ADVANCED_FACE ( 'NONE', ( #1920 ), #3098, .T. ) ;
#8449=EDGE_CURVE ( 'NONE', #11423, #1941, #2917, .T. ) ;
#8453=ORIENTED_EDGE ( 'NONE', *, *, #1611, .F. ) ;
#8455=PRODUCT ( 'Pulse _ Speed Control Dial', 'Pulse _ Speed Control Dial', '', ( #11482 ) ) ;
#8456=DIRECTION ( 'NONE',  ( -0.000000000000000000, -0.000000000000000000, 1.000000000000000000 ) ) ;
#8462=PLANE ( 'NONE',  #3551 ) ;
#8470=FACE_OUTER_BOUND ( 'NONE', #7486, .T. ) ;
#8477=VERTEX_POINT ( 'NONE', #2473 ) ;
#8484=CARTESIAN_POINT ( 'NONE',  ( -0.9407811293054709756, 43.00000000000008527, 79.50000000000000000 ) ) ;
#8485=DIRECTION ( 'NONE',  ( 0.8660254037844377084, -0.5000000000000015543, 0.000000000000000000 ) ) ;
#8489=ORIENTED_EDGE ( 'NONE', *, *, #8924, .F. ) ;
#8490=FILL_AREA_STYLE ('',( #7692 ) ) ;
#8497=ORIENTED_EDGE ( 'NONE', *, *, #865, .F. ) ;
#8501=CARTESIAN_POINT ( 'NONE',  ( 11.80921887069467324, 30.25000000000018474, 80.00000000000000000 ) ) ;
#8508=DIRECTION ( 'NONE',  ( 0.5000000000000066613, 0.8660254037844347108, 0.000000000000000000 ) ) ;
#8515=CARTESIAN_POINT ( 'NONE',  ( -12.57411137850301763, 23.71650635094618664, 79.50000000000000000 ) ) ;
#8516=CARTESIAN_POINT ( 'NONE',  ( -1.440781129305282571, 17.00000000000009592, 79.50000000000000000 ) ) ;
#8518=CARTESIAN_POINT ( 'NONE',  ( 8.809218870694669690, 29.75000000000019540, 80.00000000000000000 ) ) ;
#8521=ORIENTED_EDGE ( 'NONE', *, *, #7267, .T. ) ;
#8535=VECTOR ( 'NONE', #3670, 1000.000000000000000 ) ;
#8538=LINE ( 'NONE', #9717, #9127 ) ;
#8541=CARTESIAN_POINT ( 'NONE',  ( -5.974274778359230709, 38.78525403784446723, 80.00000000000000000 ) ) ;
#8549=DIRECTION ( 'NONE',  ( 1.000000000000000000, 0.000000000000000000, 0.000000000000000000 ) ) ;
#8553=EDGE_CURVE ( 'NONE', #4222, #10014, #2343, .T. ) ;
#8554=AXIS2_PLACEMENT_3D ( 'NONE', #3015, #7687, #8549 ) ;
#8563=LINE ( 'NONE', #8501, #11392 ) ;
#8574=ORIENTED_EDGE ( 'NONE', *, *, #844, .F. ) ;
#8583=CARTESIAN_POINT ( 'NONE',  ( -12.32411137850303184, 36.71650635094619730, 79.50000000000000000 ) ) ;
#8588=VERTEX_POINT ( 'NONE', #6275 ) ;
#8589=EDGE_CURVE ( 'NONE', #11972, #1312, #10065, .T. ) ;
#8602=LINE ( 'NONE', #5754, #7554 ) ;
#8609=ADVANCED_FACE ( 'NONE', ( #9431 ), #7276, .T. ) ;
#8612=CARTESIAN_POINT ( 'NONE',  ( -5.974274778359230709, 38.78525403784446723, 79.50000000000000000 ) ) ;
#8617=VERTEX_POINT ( 'NONE', #2716 ) ;
#8628=ORIENTED_EDGE ( 'NONE', *, *, #11133, .F. ) ;
#8629=ADVANCED_FACE ( 'NONE', ( #1842 ), #3591, .F. ) ;
#8645=EDGE_CURVE ( 'NONE', #7990, #10179, #11202, .T. ) ;
#8651=DIRECTION ( 'NONE',  ( -0.8660254037844394848, 0.4999999999999985567, 0.000000000000000000 ) ) ;
#8652=VERTEX_POINT ( 'NONE', #7517 ) ;
#8654=VECTOR ( 'NONE', #12082, 1000.000000000000114 ) ;
#8656=CIRCLE ( 'NONE', #10250, 12.99999999999999822 ) ;
#8658=CARTESIAN_POINT ( 'NONE',  ( 5.525725221640833240, 18.86666975080242992, 80.00000000000000000 ) ) ;
#8663=ORIENTED_EDGE ( 'NONE', *, *, #4806, .F. ) ;
#8679=ORIENTED_EDGE ( 'NONE', *, *, #8827, .F. ) ;
#8680=SURFACE_SIDE_STYLE ('',( #7630 ) ) ;
#8685=LINE ( 'NONE', #8867, #6892 ) ;
#8686=ORIENTED_EDGE ( 'NONE', *, *, #1176, .F. ) ;
#8699=LINE ( 'NONE', #2106, #914 ) ;
#8717=FACE_OUTER_BOUND ( 'NONE', #7721, .T. ) ;
#8720=MANIFOLD_SOLID_BREP ( 'Cut-Extrude-Thin1', #7678 ) ;
#8724=EDGE_LOOP ( 'NONE', ( #760, #3288, #9295, #5870, #1305 ) ) ;
#8725=CARTESIAN_POINT ( 'NONE',  ( -1.440781129305471087, 43.00000000000008527, 79.50000000000000000 ) ) ;
#8727=ORIENTED_EDGE ( 'NONE', *, *, #4771, .F. ) ;
#8729=CARTESIAN_POINT ( 'NONE',  ( -12.32411137850303184, 36.71650635094619730, 79.50000000000000000 ) ) ;
#8730=VERTEX_POINT ( 'NONE', #1098 ) ;
#8733=LINE ( 'NONE', #8612, #9154 ) ;
#8735=CARTESIAN_POINT ( 'NONE',  ( -9.976035167149682081, 25.21650635094616533, 80.00000000000000000 ) ) ;
#8744=ORIENTED_EDGE ( 'NONE', *, *, #6347, .T. ) ;
#8746=VECTOR ( 'NONE', #750, 1000.000000000000000 ) ;
#8753=AXIS2_PLACEMENT_3D ( 'NONE', #12052, #10095, #9980 ) ;
#8761=CIRCLE ( 'NONE', #9951, 2.000000000000001776 ) ;
#8762=LINE ( 'NONE', #1175, #10636 ) ;
#8771=EDGE_CURVE ( 'NONE', #2880, #1574, #3101, .T. ) ;
#8773=DIRECTION ( 'NONE',  ( -6.938893903907222067E-15, -1.000000000000000000, 0.000000000000000000 ) ) ;
#8775=CARTESIAN_POINT ( 'NONE',  ( -0.9407811293054709756, 40.00000000000008527, 79.50000000000000000 ) ) ;
#8778=CARTESIAN_POINT ( 'NONE',  ( 4.025725221640669815, 38.53525403784453118, 79.50000000000000000 ) ) ;
#8785=VECTOR ( 'NONE', #11899, 1000.000000000000000 ) ;
#8791=CARTESIAN_POINT ( 'NONE',  ( -7.474274778359198734, 41.38333024919781167, 80.00000000000000000 ) ) ;
#8801=LINE ( 'NONE', #11818, #885 ) ;
#8802=FACE_OUTER_BOUND ( 'NONE', #11364, .T. ) ;
#8808=EDGE_CURVE ( 'NONE', #9640, #4568, #9494, .T. ) ;
#8815=CARTESIAN_POINT ( 'NONE',  ( -1.190781129305471087, 30.00000000000008882, 80.00000000000000000 ) ) ;
#8822=ADVANCED_FACE ( 'NONE', ( #10052 ), #10997, .T. ) ;
#8827=EDGE_CURVE ( 'NONE', #4808, #3422, #8118, .T. ) ;
#8828=AXIS2_PLACEMENT_3D ( 'NONE', #10245, #2587, #3341 ) ;
#8835=VERTEX_POINT ( 'NONE', #6140 ) ;
#8840=VECTOR ( 'NONE', #5573, 1000.000000000000114 ) ;
#8847=CARTESIAN_POINT ( 'NONE',  ( 7.344472908539098732, 24.78349364905406205, 79.50000000000000000 ) ) ;
#8864=ORIENTED_EDGE ( 'NONE', *, *, #1928, .F. ) ;
#8866=CARTESIAN_POINT ( 'NONE',  ( -0.9407811293054709756, 40.00000000000008527, 80.00000000000000000 ) ) ;
#8867=CARTESIAN_POINT ( 'NONE',  ( -14.19078112930533209, 29.75000000000008882, 80.00000000000000000 ) ) ;
#8869=CARTESIAN_POINT ( 'NONE',  ( -9.976035167149682081, 25.21650635094616533, 79.50000000000000000 ) ) ;
#8875=ORIENTED_EDGE ( 'NONE', *, *, #2038, .F. ) ;
#8879=VECTOR ( 'NONE', #4569, 1000.000000000000000 ) ;
#8885=CARTESIAN_POINT ( 'NONE',  ( -7.907287480251421030, 41.13333024919781167, 80.00000000000000000 ) ) ;
#8900=EDGE_CURVE ( 'NONE', #8617, #3205, #11759, .T. ) ;
#8924=EDGE_CURVE ( 'NONE', #2786, #8477, #10238, .T. ) ;
#8927=CARTESIAN_POINT ( 'NONE',  ( -1.440781129305261477, 20.00000000000009592, 80.00000000000000000 ) ) ;
#8935=AXIS2_PLACEMENT_3D ( 'NONE', #2, #187, #1073 ) ;
#8950=VECTOR ( 'NONE', #1660, 1000.000000000000000 ) ;
#8960=ORIENTED_EDGE ( 'NONE', *, *, #832, .F. ) ;
#8973=DIRECTION ( 'NONE',  ( -0.000000000000000000, -0.000000000000000000, 1.000000000000000000 ) ) ;
#8976=VECTOR ( 'NONE', #6460, 1000.000000000000114 ) ;
#8981=ADVANCED_FACE ( 'NONE', ( #10108 ), #9235, .T. ) ;
#8991=DIRECTION ( 'NONE',  ( 0.4999999999999914513, -0.8660254037844435926, 0.000000000000000000 ) ) ;
#8993=ORIENTED_EDGE ( 'NONE', *, *, #6848, .T. ) ;
#8996=LINE ( 'NONE', #7269, #11924 ) ;
#8998=DIRECTION ( 'NONE',  ( 0.8660254037844434816, 0.4999999999999913958, 0.000000000000000000 ) ) ;
#9011=ORIENTED_EDGE ( 'NONE', *, *, #11916, .T. ) ;
#9014=ORIENTED_EDGE ( 'NONE', *, *, #9888, .T. ) ;
#9030=VERTEX_POINT ( 'NONE', #3577 ) ;
#9038=EDGE_CURVE ( 'NONE', #4568, #6913, #9296, .T. ) ;
#9042=DIRECTION ( 'NONE',  ( -0.000000000000000000, -0.000000000000000000, 1.000000000000000000 ) ) ;
#9043=PLANE ( 'NONE',  #9435 ) ;
#9044=VERTEX_POINT ( 'NONE', #7446 ) ;
#9050=DIRECTION ( 'NONE',  ( -0.8660254037844363761, 0.5000000000000038858, 0.000000000000000000 ) ) ;
#9052=VECTOR ( 'NONE', #6002, 1000.000000000000000 ) ;
#9053=EDGE_CURVE ( 'NONE', #9749, #11846, #2524, .T. ) ;
#9057=ORIENTED_EDGE ( 'NONE', *, *, #4838, .T. ) ;
#9063=CARTESIAN_POINT ( 'NONE',  ( -0.9407811293052825707, 17.00000000000008882, 79.50000000000000000 ) ) ;
#9079=DIRECTION ( 'NONE',  ( -0.000000000000000000, -1.000000000000000000, 0.000000000000000000 ) ) ;
#9094=ORIENTED_EDGE ( 'NONE', *, *, #27, .T. ) ;
#9106=CARTESIAN_POINT ( 'NONE',  ( 11.80921887069467324, 30.25000000000018474, 79.50000000000000000 ) ) ;
#9109=ADVANCED_FACE ( 'NONE', ( #899 ), #10423, .T. ) ;
#9126=AXIS2_PLACEMENT_3D ( 'NONE', #3791, #1981, #9635 ) ;
#9127=VECTOR ( 'NONE', #1197, 1000.000000000000000 ) ;
#9132=ORIENTED_EDGE ( 'NONE', *, *, #7536, .F. ) ;
#9135=ORIENTED_EDGE ( 'NONE', *, *, #11312, .T. ) ;
#9137=CARTESIAN_POINT ( 'NONE',  ( -7.474274778359198734, 41.38333024919781167, 80.00000000000000000 ) ) ;
#9142=EDGE_CURVE ( 'NONE', #10836, #3922, #1887, .T. ) ;
#9145=AXIS2_PLACEMENT_3D ( 'NONE', #9376, #7406, #10257 ) ;
#9147=CARTESIAN_POINT ( 'NONE',  ( -12.44911137850304250, 36.50000000000007816, 80.00000000000000000 ) ) ;
#9154=VECTOR ( 'NONE', #195, 1000.000000000000000 ) ;
#9155=DIRECTION ( 'NONE',  ( 0.5000000000000016653, 0.8660254037844378194, 0.000000000000000000 ) ) ;
#9159=DIRECTION ( 'NONE',  ( -1.000000000000000000, 0.000000000000000000, -0.000000000000000000 ) ) ;
#9160=CARTESIAN_POINT ( 'NONE',  ( -1.440781129305261477, 20.00000000000009592, 79.50000000000000000 ) ) ;
#9161=ADVANCED_FACE ( 'NONE', ( #3949 ), #2950, .F. ) ;
#9162=AXIS2_PLACEMENT_3D ( 'NONE', #1635, #7547, #4737 ) ;
#9168=CARTESIAN_POINT ( 'NONE',  ( -0.9407811293052825707, 17.00000000000008882, 79.50000000000000000 ) ) ;
#9169=EDGE_LOOP ( 'NONE', ( #28, #2196, #5145, #6477 ) ) ;
#9187=DIRECTION ( 'NONE',  ( -0.000000000000000000, -0.000000000000000000, 1.000000000000000000 ) ) ;
#9194=LINE ( 'NONE', #3659, #6010 ) ;
#9197=EDGE_CURVE ( 'NONE', #5363, #2747, #1829, .T. ) ;
#9201=CARTESIAN_POINT ( 'NONE',  ( 7.594472908538985045, 34.78349364905407270, 79.50000000000000000 ) ) ;
#9204=CARTESIAN_POINT ( 'NONE',  ( -0.9407811293052825707, 17.00000000000008882, 79.50000000000000000 ) ) ;
#9212=ORIENTED_EDGE ( 'NONE', *, *, #11763, .F. ) ;
#9218=CARTESIAN_POINT ( 'NONE',  ( -1.440781129305471087, 43.00000000000008527, 79.50000000000000000 ) ) ;
#9223=CARTESIAN_POINT ( 'NONE',  ( 9.942549119892305498, 36.71650635094628967, 80.00000000000000000 ) ) ;
#9224=ORIENTED_EDGE ( 'NONE', *, *, #1079, .T. ) ;
#9227=VECTOR ( 'NONE', #4629, 999.9999999999998863 ) ;
#9234=EDGE_CURVE ( 'NONE', #1251, #9416, #11927, .T. ) ;
#9235=PLANE ( 'NONE',  #11297 ) ;
#9239=AXIS2_PLACEMENT_3D ( 'NONE', #2120, #11351, #11413 ) ;
#9240=ORIENTED_EDGE ( 'NONE', *, *, #6953, .F. ) ;
#9242=VECTOR ( 'NONE', #6809, 1000.000000000000000 ) ;
#9244=CARTESIAN_POINT ( 'NONE',  ( 13.80921887069452758, 30.00000000000008882, 78.00000000000000000 ) ) ;
#9247=CARTESIAN_POINT ( 'NONE',  ( 4.025725221640849227, 21.46474596215575659, 79.50000000000000000 ) ) ;
#9264=ORIENTED_EDGE ( 'NONE', *, *, #9888, .F. ) ;
#9268=EDGE_CURVE ( 'NONE', #10198, #2842, #1264, .T. ) ;
#9275=ORIENTED_EDGE ( 'NONE', *, *, #9234, .T. ) ;
#9279=ORIENTED_EDGE ( 'NONE', *, *, #9053, .F. ) ;
#9282=SHAPE_REPRESENTATION_RELATIONSHIP ( 'NONE' , 'NONE' ,  #12244, #11672 ) ;
#9289=ORIENTED_EDGE ( 'NONE', *, *, #953, .F. ) ;
#9292=ORIENTED_EDGE ( 'NONE', *, *, #4621, .T. ) ;
#9295=ORIENTED_EDGE ( 'NONE', *, *, #2819, .F. ) ;
#9296=LINE ( 'NONE', #783, #8879 ) ;
#9297=LINE ( 'NONE', #4756, #8161 ) ;
#9310=CARTESIAN_POINT ( 'NONE',  ( -11.19078112930532853, 29.75000000000005684, 79.50000000000000000 ) ) ;
#9316=DIRECTION ( 'NONE',  ( -0.4999999999999985012, 0.8660254037844394848, 0.000000000000000000 ) ) ;
#9318=DIRECTION ( 'NONE',  ( 0.4999999999999878431, -0.8660254037844455910, 0.000000000000000000 ) ) ;
#9320=DIRECTION ( 'NONE',  ( 0.8660254037844385966, -0.5000000000000000000, 0.000000000000000000 ) ) ;
#9321=PLANE ( 'NONE',  #2282 ) ;
#9323=VERTEX_POINT ( 'NONE', #2252 ) ;
#9325=DIRECTION ( 'NONE',  ( 6.938893903907222067E-15, 1.000000000000000000, 0.000000000000000000 ) ) ;
#9326=VECTOR ( 'NONE', #11637, 1000.000000000000000 ) ;
#9333=CARTESIAN_POINT ( 'NONE',  ( -14.19078112930532853, 30.25000000000008882, 80.00000000000000000 ) ) ;
#9337=DIRECTION ( 'NONE',  ( -0.8660254037844424824, -0.4999999999999933387, 0.000000000000000000 ) ) ;
#9338=EDGE_LOOP ( 'NONE', ( #4687, #9240, #925, #4604, #10852 ) ) ;
#9341=PLANE ( 'NONE',  #5407 ) ;
#9347=ORIENTED_EDGE ( 'NONE', *, *, #1655, .T. ) ;
#9349=CARTESIAN_POINT ( 'NONE',  ( 4.025725221640669815, 38.53525403784453118, 79.50000000000000000 ) ) ;
#9356=VECTOR ( 'NONE', #10439, 1000.000000000000114 ) ;
#9360=LINE ( 'NONE', #6281, #9454 ) ;
#9371=DIRECTION ( 'NONE',  ( -0.000000000000000000, -0.000000000000000000, -1.000000000000000000 ) ) ;
#9376=CARTESIAN_POINT ( 'NONE',  ( 11.80921887069467324, 29.75000000000018474, 79.50000000000000000 ) ) ;
#9382=DIRECTION ( 'NONE',  ( 1.000000000000000000, 0.000000000000000000, 0.000000000000000000 ) ) ;
#9403=ORIENTED_EDGE ( 'NONE', *, *, #6863, .F. ) ;
#9406=EDGE_CURVE ( 'NONE', #11096, #4895, #4431, .T. ) ;
#9408=ADVANCED_FACE ( 'NONE', ( #2626 ), #698, .T. ) ;
#9412=VERTEX_POINT ( 'NONE', #8162 ) ;
#9414=CARTESIAN_POINT ( 'NONE',  ( 5.525725221640672480, 41.13333024919784719, 80.00000000000000000 ) ) ;
#9415=VECTOR ( 'NONE', #4275, 1000.000000000000114 ) ;
#9416=VERTEX_POINT ( 'NONE', #8411 ) ;
#9431=FACE_OUTER_BOUND ( 'NONE', #1810, .T. ) ;
#9435=AXIS2_PLACEMENT_3D ( 'NONE', #4439, #7253, #10103 ) ;
#9438=AXIS2_PLACEMENT_3D ( 'NONE', #6108, #488, #5172 ) ;
#9450=CARTESIAN_POINT ( 'NONE',  ( -1.190781129305471087, 30.00000000000008882, 80.00000000000000000 ) ) ;
#9453=PLANE ( 'NONE',  #1000 ) ;
#9454=VECTOR ( 'NONE', #12311, 1000.000000000000000 ) ;
#9460=ORIENTED_EDGE ( 'NONE', *, *, #7083, .F. ) ;
#9463=DIRECTION ( 'NONE',  ( -1.000000000000000000, 0.000000000000000000, 0.000000000000000000 ) ) ;
#9469=DIRECTION ( 'NONE',  ( 0.000000000000000000, -1.000000000000000000, 0.000000000000000000 ) ) ;
#9472=CARTESIAN_POINT ( 'NONE',  ( -12.57411137850301763, 23.71650635094618664, 79.50000000000000000 ) ) ;
#9473=STYLED_ITEM ( 'NONE', ( #2964 ), #8720 ) ;
#9475=CARTESIAN_POINT ( 'NONE',  ( 10.19254911989230727, 36.28349364905406560, 79.50000000000000000 ) ) ;
#9476=FACE_OUTER_BOUND ( 'NONE', #8345, .T. ) ;
#9479=FACE_OUTER_BOUND ( 'NONE', #8724, .T. ) ;
#9482=CARTESIAN_POINT ( 'NONE',  ( 11.80921887069467324, 29.75000000000018474, 79.50000000000000000 ) ) ;
#9485=LINE ( 'NONE', #3354, #2504 ) ;
#9486=ORIENTED_EDGE ( 'NONE', *, *, #11242, .F. ) ;
#9488=CARTESIAN_POINT ( 'NONE',  ( -1.190781129305471087, 30.00000000000008882, 80.00000000000000000 ) ) ;
#9494=LINE ( 'NONE', #10503, #3312 ) ;
#9509=DIRECTION ( 'NONE',  ( 0.8660254037844434816, 0.4999999999999913958, 0.000000000000000000 ) ) ;
#9514=AXIS2_PLACEMENT_3D ( 'NONE', #4875, #5689, #7795 ) ;
#9516=ORIENTED_EDGE ( 'NONE', *, *, #10096, .F. ) ;
#9517=FACE_OUTER_BOUND ( 'NONE', #9548, .T. ) ;
#9522=ORIENTED_EDGE ( 'NONE', *, *, #6837, .F. ) ;
#9526=DIRECTION ( 'NONE',  ( -0.000000000000000000, -0.000000000000000000, 1.000000000000000000 ) ) ;
#9532=AXIS2_PLACEMENT_3D ( 'NONE', #2111, #10459, #4723 ) ;
#9533=AXIS2_PLACEMENT_3D ( 'NONE', #7378, #3514, #6318 ) ;
#9536=CARTESIAN_POINT ( 'NONE',  ( -1.190781129305471087, 30.00000000000008882, 80.00000000000000000 ) ) ;
#9548=EDGE_LOOP ( 'NONE', ( #5358, #9279, #11861, #4760, #2383 ) ) ;
#9562=CARTESIAN_POINT ( 'NONE',  ( 0.000000000000000000, 0.000000000000000000, 0.000000000000000000 ) ) ;
#9565=VECTOR ( 'NONE', #11586, 1000.000000000000000 ) ;
#9573=VERTEX_POINT ( 'NONE', #7546 ) ;
#9575=CARTESIAN_POINT ( 'NONE',  ( -7.690781129305409358, 41.25833024919774772, 80.00000000000000000 ) ) ;
#9576=VECTOR ( 'NONE', #8998, 1000.000000000000114 ) ;
#9580=EDGE_CURVE ( 'NONE', #10794, #9030, #883, .T. ) ;
#9582=ORIENTED_EDGE ( 'NONE', *, *, #7217, .F. ) ;
#9588=VERTEX_POINT ( 'NONE', #3869 ) ;
#9589=DIRECTION ( 'NONE',  ( 0.000000000000000000, 0.000000000000000000, 1.000000000000000000 ) ) ;
#9591=CARTESIAN_POINT ( 'NONE',  ( 5.092712519748452848, 41.38333024919784719, 79.50000000000000000 ) ) ;
#9594=EDGE_LOOP ( 'NONE', ( #9486, #4440, #779, #8248, #2357 ) ) ;
#9597=VECTOR ( 'NONE', #5149, 1000.000000000000000 ) ;
#9598=ORIENTED_EDGE ( 'NONE', *, *, #277, .F. ) ;
#9601=ORIENTED_EDGE ( 'NONE', *, *, #10274, .T. ) ;
#9606=DIRECTION ( 'NONE',  ( 1.000000000000000000, -1.040834085586083310E-14, 0.000000000000000000 ) ) ;
#9607=DIRECTION ( 'NONE',  ( -1.000000000000000000, 0.000000000000000000, -0.000000000000000000 ) ) ;
#9613=LINE ( 'NONE', #392, #7452 ) ;
#9615=DIRECTION ( 'NONE',  ( -0.5000000000000005551, -0.8660254037844382635, 0.000000000000000000 ) ) ;
#9633=ORIENTED_EDGE ( 'NONE', *, *, #6942, .T. ) ;
#9635=DIRECTION ( 'NONE',  ( 1.000000000000000000, 0.000000000000000000, 0.000000000000000000 ) ) ;
#9640=VERTEX_POINT ( 'NONE', #2659 ) ;
#9641=DIRECTION ( 'NONE',  ( -0.8660254037844398178, -0.4999999999999977796, 0.000000000000000000 ) ) ;
#9643=ORIENTED_EDGE ( 'NONE', *, *, #9809, .F. ) ;
#9650=DIRECTION ( 'NONE',  ( 1.000000000000000000, 0.000000000000000000, 0.000000000000000000 ) ) ;
#9656=EDGE_LOOP ( 'NONE', ( #3374, #8489, #8001, #11716 ) ) ;
#9658=LINE ( 'NONE', #9475, #1389 ) ;
#9659=EDGE_CURVE ( 'NONE', #9755, #4568, #4578, .T. ) ;
#9663=CARTESIAN_POINT ( 'NONE',  ( -9.726035167149685634, 24.78349364905394125, 79.50000000000000000 ) ) ;
#9664=DIRECTION ( 'NONE',  ( 0.4999999999999877875, -0.8660254037844457020, 0.000000000000000000 ) ) ;
#9673=EDGE_CURVE ( 'NONE', #7589, #6190, #9194, .T. ) ;
#9679=LINE ( 'NONE', #10373, #10601 ) ;
#9684=EDGE_LOOP ( 'NONE', ( #401, #3499, #315, #11909, #5118 ) ) ;
#9692=DIRECTION ( 'NONE',  ( 1.000000000000000000, -7.011174048739587977E-15, 0.000000000000000000 ) ) ;
#9699=ORIENTED_EDGE ( 'NONE', *, *, #7521, .F. ) ;
#9709=DIRECTION ( 'NONE',  ( 1.000000000000000000, 0.000000000000000000, 0.000000000000000000 ) ) ;
#9714=EDGE_CURVE ( 'NONE', #8835, #5671, #5352, .T. ) ;
#9717=CARTESIAN_POINT ( 'NONE',  ( -7.474274778359198734, 41.38333024919781167, 79.50000000000000000 ) ) ;
#9719=ORIENTED_EDGE ( 'NONE', *, *, #10254, .T. ) ;
#9725=CARTESIAN_POINT ( 'NONE',  ( 0.000000000000000000, 0.000000000000000000, 79.50000000000000000 ) ) ;
#9726=VECTOR ( 'NONE', #6269, 1000.000000000000000 ) ;
#9727=LINE ( 'NONE', #1207, #11352 ) ;
#9741=CARTESIAN_POINT ( 'NONE',  ( -12.40744471183567299, 36.57216878364999246, 80.00000000000000000 ) ) ;
#9744=EDGE_CURVE ( 'NONE', #8617, #867, #11137, .T. ) ;
#9749=VERTEX_POINT ( 'NONE', #3414 ) ;
#9751=B_SPLINE_CURVE_WITH_KNOTS ( 'NONE', 3,
 ( #1823, #4564, #6441, #10230 ),
 .UNSPECIFIED., .F., .F.,
 ( 4, 4 ),
 ( 0.0009573067811869144170, 0.001207306781186545577 ),
 .UNSPECIFIED. ) ;
#9754=PLANE ( 'NONE',  #6209 ) ;
#9755=VERTEX_POINT ( 'NONE', #6276 ) ;
#9757=DIRECTION ( 'NONE',  ( -0.8660254037844383745, 0.5000000000000006661, 0.000000000000000000 ) ) ;
#9763=ORIENTED_EDGE ( 'NONE', *, *, #3275, .T. ) ;
#9764=CARTESIAN_POINT ( 'NONE',  ( -12.32411137850303184, 36.71650635094619730, 80.00000000000000000 ) ) ;
#9767=CARTESIAN_POINT ( 'NONE',  ( -11.19078112930532498, 30.25000000000005684, 80.00000000000000000 ) ) ;
#9768=ORIENTED_EDGE ( 'NONE', *, *, #10770, .T. ) ;
#9775=VECTOR ( 'NONE', #3597, 1000.000000000000000 ) ;
#9776=CARTESIAN_POINT ( 'NONE',  ( -7.474274778359196070, 18.61666975080236597, 80.00000000000000000 ) ) ;
#9785=LINE ( 'NONE', #9663, #6598 ) ;
#9786=CARTESIAN_POINT ( 'NONE',  ( -1.440781129305471087, 43.00000000000008527, 80.00000000000000000 ) ) ;
#9795=AXIS2_PLACEMENT_3D ( 'NONE', #5741, #4381, #9463 ) ;
#9801=DIRECTION ( 'NONE',  ( 0.8660254037844377084, -0.5000000000000015543, 0.000000000000000000 ) ) ;
#9804=CARTESIAN_POINT ( 'NONE',  ( 5.309218870694537351, 18.74166975080233044, 80.00000000000000000 ) ) ;
#9809=EDGE_CURVE ( 'NONE', #5368, #3755, #3350, .T. ) ;
#9816=LINE ( 'NONE', #8071, #1504 ) ;
#9823=DIRECTION ( 'NONE',  ( -0.8660254037844399289, -0.4999999999999977796, 0.000000000000000000 ) ) ;
#9827=CARTESIAN_POINT ( 'NONE',  ( -12.32411137850302119, 23.28349364905396612, 79.50000000000000000 ) ) ;
#9840=ORIENTED_EDGE ( 'NONE', *, *, #2567, .F. ) ;
#9846=AXIS2_PLACEMENT_3D ( 'NONE', #8039, #3378, #10979 ) ;
#9849=ORIENTED_EDGE ( 'NONE', *, *, #10513, .T. ) ;
#9860=PLANE ( 'NONE',  #6471 ) ;
#9875=EDGE_LOOP ( 'NONE', ( #8271, #1320, #6495, #9633, #1505 ) ) ;
#9887=EDGE_CURVE ( 'NONE', #12341, #3922, #7577, .T. ) ;
#9888=EDGE_CURVE ( 'NONE', #828, #10546, #8382, .T. ) ;
#9891=CARTESIAN_POINT ( 'NONE',  ( 7.594472908538985045, 34.78349364905407270, 79.50000000000000000 ) ) ;
#9903=EDGE_CURVE ( 'NONE', #9573, #11089, #8563, .T. ) ;
#9904=ORIENTED_EDGE ( 'NONE', *, *, #997, .F. ) ;
#9907=ORIENTED_EDGE ( 'NONE', *, *, #8589, .T. ) ;
#9909=CARTESIAN_POINT ( 'NONE',  ( -9.726035167149728267, 35.21650635094616888, 79.50000000000000000 ) ) ;
#9910=VERTEX_POINT ( 'NONE', #3654 ) ;
#9922=DIRECTION ( 'NONE',  ( -0.5000000000000006661, -0.8660254037844383745, 0.000000000000000000 ) ) ;
#9930=CARTESIAN_POINT ( 'NONE',  ( 9.942549119892413856, 23.28349364905404428, 79.50000000000000000 ) ) ;
#9931=FACE_OUTER_BOUND ( 'NONE', #5240, .T. ) ;
#9932=ORIENTED_EDGE ( 'NONE', *, *, #3703, .T. ) ;
#9938=CARTESIAN_POINT ( 'NONE',  ( -12.57411137850301763, 23.71650635094618664, 79.50000000000000000 ) ) ;
#9949=ADVANCED_FACE ( 'NONE', ( #10377 ), #7461, .T. ) ;
#9950=ORIENTED_EDGE ( 'NONE', *, *, #9197, .F. ) ;
#9951=AXIS2_PLACEMENT_3D ( 'NONE', #6037, #11015, #10950 ) ;
#9961=ORIENTED_EDGE ( 'NONE', *, *, #323, .T. ) ;
#9965=ORIENTED_EDGE ( 'NONE', *, *, #1779, .T. ) ;
#9980=DIRECTION ( 'NONE',  ( 1.000000000000000000, 0.000000000000000000, 0.000000000000000000 ) ) ;
#9986=LINE ( 'NONE', #2325, #1291 ) ;
#9987=ORIENTED_EDGE ( 'NONE', *, *, #1907, .F. ) ;
#10006=LINE ( 'NONE', #11077, #5891 ) ;
#10014=VERTEX_POINT ( 'NONE', #150 ) ;
#10015=VECTOR ( 'NONE', #11397, 1000.000000000000000 ) ;
#10016=CARTESIAN_POINT ( 'NONE',  ( -0.9407811293054709756, 42.99759593155604875, 80.00000000000000000 ) ) ;
#10026=VECTOR ( 'NONE', #7331, 1000.000000000000114 ) ;
#10029=LINE ( 'NONE', #4063, #355 ) ;
#10032=VERTEX_POINT ( 'NONE', #213 ) ;
#10044=EDGE_LOOP ( 'NONE', ( #9768, #352, #1916, #7845, #4319 ) ) ;
#10051=CARTESIAN_POINT ( 'NONE',  ( 5.091510485526399954, 41.38124826485281460, 80.00000000000000000 ) ) ;
#10052=FACE_OUTER_BOUND ( 'NONE', #10774, .T. ) ;
#10061=DIRECTION ( 'NONE',  ( 1.000000000000000000, -1.040834085586083310E-14, 0.000000000000000000 ) ) ;
#10062=CARTESIAN_POINT ( 'NONE',  ( -1.440781129305282571, 17.00000000000009592, 80.00000000000000000 ) ) ;
#10065=LINE ( 'NONE', #2225, #3117 ) ;
#10070=CARTESIAN_POINT ( 'NONE',  ( -14.19078112930532853, 30.25000000000008882, 80.00000000000000000 ) ) ;
#10083=DIRECTION ( 'NONE',  ( -0.8660254037844457020, -0.4999999999999877875, 0.000000000000000000 ) ) ;
#10088=CARTESIAN_POINT ( 'NONE',  ( 5.525725221640833240, 18.86666975080242992, 79.50000000000000000 ) ) ;
#10090=ORIENTED_EDGE ( 'NONE', *, *, #7765, .F. ) ;
#10093=CARTESIAN_POINT ( 'NONE',  ( -12.44911137850311000, 23.50000000000024158, 80.00000000000000000 ) ) ;
#10095=DIRECTION ( 'NONE',  ( 0.000000000000000000, 0.000000000000000000, 1.000000000000000000 ) ) ;
#10096=EDGE_CURVE ( 'NONE', #7629, #872, #10627, .T. ) ;
#10099=ORIENTED_EDGE ( 'NONE', *, *, #2719, .T. ) ;
#10103=DIRECTION ( 'NONE',  ( 0.8660254037844399289, 0.4999999999999977796, 0.000000000000000000 ) ) ;
#10108=FACE_OUTER_BOUND ( 'NONE', #9338, .T. ) ;
#10114=ORIENTED_EDGE ( 'NONE', *, *, #3072, .T. ) ;
#10118=CARTESIAN_POINT ( 'NONE',  ( -16.19078112930547064, 30.00000000000008882, 80.00000000000000000 ) ) ;
#10129=LINE ( 'NONE', #10193, #4188 ) ;
#10143=AXIS2_PLACEMENT_3D ( 'NONE', #73, #2017, #3951 ) ;
#10151=DIRECTION ( 'NONE',  ( 0.5000000000000038858, 0.8660254037844363761, 0.000000000000000000 ) ) ;
#10154=ADVANCED_FACE ( 'NONE', ( #9931 ), #3398, .F. ) ;
#10167=LINE ( 'NONE', #9349, #1983 ) ;
#10172=ORIENTED_EDGE ( 'NONE', *, *, #6635, .F. ) ;
#10179=VERTEX_POINT ( 'NONE', #11187 ) ;
#10184=EDGE_CURVE ( 'NONE', #10179, #1960, #8307, .T. ) ;
#10191=VERTEX_POINT ( 'NONE', #4691 ) ;
#10193=CARTESIAN_POINT ( 'NONE',  ( 7.594472908538985045, 34.78349364905407270, 80.00000000000000000 ) ) ;
#10196=ADVANCED_FACE ( 'NONE', ( #1830 ), #10489, .T. ) ;
#10198=VERTEX_POINT ( 'NONE', #5640 ) ;
#10202=EDGE_LOOP ( 'NONE', ( #6505, #6790, #10387, #7247, #3901 ) ) ;
#10205=LINE ( 'NONE', #11340, #5962 ) ;
#10225=EDGE_CURVE ( 'NONE', #2329, #8617, #9297, .T. ) ;
#10230=CARTESIAN_POINT ( 'NONE',  ( -1.440781129305282571, 17.00000000000009592, 80.00000000000000000 ) ) ;
#10233=ORIENTED_EDGE ( 'NONE', *, *, #1779, .F. ) ;
#10238=LINE ( 'NONE', #12065, #3716 ) ;
#10239=DIRECTION ( 'NONE',  ( -0.5000000000000036637, -0.8660254037844364872, 0.000000000000000000 ) ) ;
#10243=ORIENTED_EDGE ( 'NONE', *, *, #4698, .T. ) ;
#10245=CARTESIAN_POINT ( 'NONE',  ( -11.19078112930532498, 30.25000000000005684, 79.50000000000000000 ) ) ;
#10250=AXIS2_PLACEMENT_3D ( 'NONE', #5865, #9589, #9650 ) ;
#10254=EDGE_CURVE ( 'NONE', #6198, #12042, #3759, .T. ) ;
#10255=EDGE_LOOP ( 'NONE', ( #2352, #5848, #37, #7255, #6834 ) ) ;
#10257=DIRECTION ( 'NONE',  ( -1.000000000000000000, 3.469446951953611033E-15, 0.000000000000000000 ) ) ;
#10269=CARTESIAN_POINT ( 'NONE',  ( 5.525725221640833240, 18.86666975080242992, 80.00000000000000000 ) ) ;
#10274=EDGE_CURVE ( 'NONE', #3881, #3399, #11, .T. ) ;
#10280=DIRECTION ( 'NONE',  ( 0.4999999999999981681, -0.8660254037844397068, 0.000000000000000000 ) ) ;
#10287=EDGE_CURVE ( 'NONE', #9749, #9910, #4570, .T. ) ;
#10298=ORIENTED_EDGE ( 'NONE', *, *, #11128, .T. ) ;
#10302=LINE ( 'NONE', #10070, #7282 ) ;
#10321=FACE_OUTER_BOUND ( 'NONE', #806, .T. ) ;
#10322=CARTESIAN_POINT ( 'NONE',  ( 11.80921887069467324, 30.00000000000008882, 80.00000000000000000 ) ) ;
#10324=EDGE_CURVE ( 'NONE', #10014, #10191, #6063, .T. ) ;
#10327=CARTESIAN_POINT ( 'NONE',  ( -14.19078112930533209, 29.75000000000008882, 79.50000000000000000 ) ) ;
#10331=EDGE_LOOP ( 'NONE', ( #5078, #3020, #11481, #10692, #9094 ) ) ;
#10338=ORIENTED_EDGE ( 'NONE', *, *, #6254, .T. ) ;
#10340=ADVANCED_FACE ( 'NONE', ( #11624 ), #135, .F. ) ;
#10345=ORIENTED_EDGE ( 'NONE', *, *, #844, .T. ) ;
#10351=ORIENTED_EDGE ( 'NONE', *, *, #8093, .T. ) ;
#10355=DIRECTION ( 'NONE',  ( 0.000000000000000000, 0.000000000000000000, 1.000000000000000000 ) ) ;
#10358=DIRECTION ( 'NONE',  ( -0.5000000000000006661, -0.8660254037844383745, 0.000000000000000000 ) ) ;
#10371=ORIENTED_EDGE ( 'NONE', *, *, #10472, .F. ) ;
#10373=CARTESIAN_POINT ( 'NONE',  ( -12.32411137850302119, 23.28349364905396612, 80.00000000000000000 ) ) ;
#10377=FACE_OUTER_BOUND ( 'NONE', #3165, .T. ) ;
#10379=EDGE_CURVE ( 'NONE', #11969, #5385, #2016, .T. ) ;
#10381=VECTOR ( 'NONE', #1539, 1000.000000000000000 ) ;
#10382=VECTOR ( 'NONE', #6645, 1000.000000000000000 ) ;
#10384=EDGE_CURVE ( 'NONE', #5570, #6190, #8733, .T. ) ;
#10386=CARTESIAN_POINT ( 'NONE',  ( -14.19078112930532853, 30.25000000000008882, 79.50000000000000000 ) ) ;
#10387=ORIENTED_EDGE ( 'NONE', *, *, #3141, .T. ) ;
#10388=DIRECTION ( 'NONE',  ( -0.000000000000000000, -0.000000000000000000, 1.000000000000000000 ) ) ;
#10393=DIRECTION ( 'NONE',  ( -1.000000000000000000, 0.000000000000000000, -0.000000000000000000 ) ) ;
#10398=AXIS2_PLACEMENT_3D ( 'NONE', #4796, #4107, #4050 ) ;
#10399=CARTESIAN_POINT ( 'NONE',  ( 11.80681480225048752, 29.75000000000018474, 80.00000000000000000 ) ) ;
#10407=DIRECTION ( 'NONE',  ( -0.000000000000000000, -0.000000000000000000, 1.000000000000000000 ) ) ;
#10408=FACE_OUTER_BOUND ( 'NONE', #9594, .T. ) ;
#10409=EDGE_CURVE ( 'NONE', #9640, #12119, #6878, .T. ) ;
#10414=EDGE_CURVE ( 'NONE', #65, #5951, #2140, .T. ) ;
#10423=PLANE ( 'NONE',  #3123 ) ;
#10425=APPLICATION_CONTEXT ( 'automotive_design' ) ;
#10430=ADVANCED_FACE ( 'NONE', ( #2195 ), #1265, .F. ) ;
#10437=ORIENTED_EDGE ( 'NONE', *, *, #2273, .F. ) ;
#10439=DIRECTION ( 'NONE',  ( 0.5000000000000066613, 0.8660254037844347108, 0.000000000000000000 ) ) ;
#10443=AXIS2_PLACEMENT_3D ( 'NONE', #9536, #777, #4508 ) ;
#10450=LINE ( 'NONE', #11644, #4851 ) ;
#10459=DIRECTION ( 'NONE',  ( 0.000000000000000000, -1.000000000000000000, 0.000000000000000000 ) ) ;
#10470=VECTOR ( 'NONE', #11864, 1000.000000000000000 ) ;
#10472=EDGE_CURVE ( 'NONE', #11969, #12341, #8226, .T. ) ;
#10479=EDGE_LOOP ( 'NONE', ( #5293, #9212 ) ) ;
#10483=DIRECTION ( 'NONE',  ( -0.8660254037844398178, -0.4999999999999977796, 0.000000000000000000 ) ) ;
#10487=VERTEX_POINT ( 'NONE', #10093 ) ;
#10489=PLANE ( 'NONE',  #410 ) ;
#10490=ADVANCED_FACE ( 'NONE', ( #2375 ), #2564, .F. ) ;
#10493=VECTOR ( 'NONE', #7244, 1000.000000000000000 ) ;
#10499=DIRECTION ( 'NONE',  ( -0.8660254037844383745, 0.5000000000000006661, 0.000000000000000000 ) ) ;
#10501=CARTESIAN_POINT ( 'NONE',  ( 10.19254911989241386, 23.71650635094626836, 79.50000000000000000 ) ) ;
#10503=CARTESIAN_POINT ( 'NONE',  ( -0.9407811293054709756, 43.00000000000008527, 79.50000000000000000 ) ) ;
#10513=EDGE_CURVE ( 'NONE', #2786, #8835, #7310, .T. ) ;
#10514=DIRECTION ( 'NONE',  ( -0.000000000000000000, -0.000000000000000000, 1.000000000000000000 ) ) ;
#10515=PLANE ( 'NONE',  #6007 ) ;
#10517=CARTESIAN_POINT ( 'NONE',  ( 5.525725221640672480, 41.13333024919784719, 79.50000000000000000 ) ) ;
#10519=FACE_OUTER_BOUND ( 'NONE', #10479, .T. ) ;
#10521=EDGE_LOOP ( 'NONE', ( #4783, #8286, #6105, #2360, #6966 ) ) ;
#10527=DIRECTION ( 'NONE',  ( -1.000000000000000000, 0.000000000000000000, 0.000000000000000000 ) ) ;
#10535=FACE_OUTER_BOUND ( 'NONE', #5874, .T. ) ;
#10544=CARTESIAN_POINT ( 'NONE',  ( 10.06754911989234635, 23.50000000000004974, 80.00000000000000000 ) ) ;
#10545=PLANE ( 'NONE',  #7081 ) ;
#10546=VERTEX_POINT ( 'NONE', #1511 ) ;
#10561=DIRECTION ( 'NONE',  ( 0.8660254037844434816, 0.4999999999999913958, 0.000000000000000000 ) ) ;
#10565=ORIENTED_EDGE ( 'NONE', *, *, #596, .F. ) ;
#10577=CARTESIAN_POINT ( 'NONE',  ( -0.9407811293054709756, 43.00000000000008527, 80.00000000000000000 ) ) ;
#10583=VERTEX_POINT ( 'NONE', #2318 ) ;
#10601=VECTOR ( 'NONE', #10561, 1000.000000000000114 ) ;
#10602=VERTEX_POINT ( 'NONE', #10916 ) ;
#10612=DIRECTION ( 'NONE',  ( -0.000000000000000000, 0.000000000000000000, 1.000000000000000000 ) ) ;
#10613=CARTESIAN_POINT ( 'NONE',  ( 0.000000000000000000, 0.000000000000000000, 79.50000000000000000 ) ) ;
#10618=SURFACE_STYLE_USAGE ( .BOTH. , #8680 ) ;
#10627=LINE ( 'NONE', #6952, #11576 ) ;
#10634=CARTESIAN_POINT ( 'NONE',  ( 9.942549119892305498, 36.71650635094628967, 79.50000000000000000 ) ) ;
#10635=ORIENTED_EDGE ( 'NONE', *, *, #10414, .T. ) ;
#10636=VECTOR ( 'NONE', #11467, 1000.000000000000000 ) ;
#10641=LINE ( 'NONE', #40, #4357 ) ;
#10656=DIRECTION ( 'NONE',  ( 0.000000000000000000, 0.000000000000000000, 1.000000000000000000 ) ) ;
#10658=ADVANCED_FACE ( 'NONE', ( #4679 ), #9341, .T. ) ;
#10665=DIRECTION ( 'NONE',  ( -1.000000000000000000, 3.469446951953611033E-15, 0.000000000000000000 ) ) ;
#10676=DIRECTION ( 'NONE',  ( 0.000000000000000000, 0.000000000000000000, -1.000000000000000000 ) ) ;
#10692=ORIENTED_EDGE ( 'NONE', *, *, #9234, .F. ) ;
#10693=ADVANCED_FACE ( 'NONE', ( #10408 ), #7433, .T. ) ;
#10710=EDGE_LOOP ( 'NONE', ( #1270, #9460, #9601, #4854 ) ) ;
#10718=VERTEX_POINT ( 'NONE', #5626 ) ;
#10722=ADVANCED_FACE ( 'NONE', ( #8470 ), #884, .T. ) ;
#10741=LINE ( 'NONE', #3389, #4278 ) ;
#10743=PRODUCT_DEFINITION_CONTEXT ( 'detailed design', #6138, 'design' ) ;
#10759=CARTESIAN_POINT ( 'NONE',  ( -12.57411137850301763, 23.71650635094618664, 79.50000000000000000 ) ) ;
#10761=VECTOR ( 'NONE', #3889, 1000.000000000000000 ) ;
#10770=EDGE_CURVE ( 'NONE', #10718, #10032, #3935, .T. ) ;
#10774=EDGE_LOOP ( 'NONE', ( #11630, #8628, #8309, #5635, #10172 ) ) ;
#10775=PLANE ( 'NONE',  #9438 ) ;
#10779=VECTOR ( 'NONE', #9187, 1000.000000000000000 ) ;
#10782=ORIENTED_EDGE ( 'NONE', *, *, #6203, .F. ) ;
#10784=ORIENTED_EDGE ( 'NONE', *, *, #1551, .F. ) ;
#10793=CARTESIAN_POINT ( 'NONE',  ( -0.9407811293054709756, 43.00000000000008527, 79.50000000000000000 ) ) ;
#10794=VERTEX_POINT ( 'NONE', #3058 ) ;
#10805=VECTOR ( 'NONE', #110, 1000.000000000000114 ) ;
#10812=EDGE_CURVE ( 'NONE', #3922, #1521, #11609, .T. ) ;
#10826=ORIENTED_EDGE ( 'NONE', *, *, #11085, .T. ) ;
#10827=LINE ( 'NONE', #4402, #1605 ) ;
#10836=VERTEX_POINT ( 'NONE', #9591 ) ;
#10843=ORIENTED_EDGE ( 'NONE', *, *, #7016, .F. ) ;
#10852=ORIENTED_EDGE ( 'NONE', *, *, #8771, .F. ) ;
#10854=CARTESIAN_POINT ( 'NONE',  ( 10.19254911989241386, 23.71650635094626836, 80.00000000000000000 ) ) ;
#10867=EDGE_LOOP ( 'NONE', ( #11779, #6145, #10371, #2547 ) ) ;
#10869=PLANE ( 'NONE',  #5034 ) ;
#10876=( GEOMETRIC_REPRESENTATION_CONTEXT ( 3 ) GLOBAL_UNCERTAINTY_ASSIGNED_CONTEXT ( ( #8124 ) ) GLOBAL_UNIT_ASSIGNED_CONTEXT ( ( #7701, #4769, #5027 ) ) REPRESENTATION_CONTEXT ( 'NONE', 'WORKASPACE' ) );
#10881=CARTESIAN_POINT ( 'NONE',  ( 10.15088245323607907, 36.35566243268468867, 80.00000048127353125 ) ) ;
#10882=EDGE_CURVE ( 'NONE', #11846, #2311, #4870, .T. ) ;
#10890=EDGE_LOOP ( 'NONE', ( #3292, #11725, #6926, #11454 ) ) ;
#10894=ORIENTED_EDGE ( 'NONE', *, *, #6485, .T. ) ;
#10896=VERTEX_POINT ( 'NONE', #2359 ) ;
#10900=CARTESIAN_POINT ( 'NONE',  ( -12.32411137850303184, 36.71650635094619730, 79.50000000000000000 ) ) ;
#10909=DIRECTION ( 'NONE',  ( 0.4999999999999878431, -0.8660254037844455910, 0.000000000000000000 ) ) ;
#10913=STYLED_ITEM ( 'NONE', ( #2023 ), #11672 ) ;
#10916=CARTESIAN_POINT ( 'NONE',  ( 7.594472908539098732, 25.21650635094628257, 80.00000000000000000 ) ) ;
#10922=ORIENTED_EDGE ( 'NONE', *, *, #997, .T. ) ;
#10924=DIRECTION ( 'NONE',  ( -1.387778780781445676E-14, -1.000000000000000000, 0.000000000000000000 ) ) ;
#10929=DIRECTION ( 'NONE',  ( -0.5000000000000095479, -0.8660254037844331565, 0.000000000000000000 ) ) ;
#10935=ORIENTED_EDGE ( 'NONE', *, *, #3046, .F. ) ;
#10948=AXIS2_PLACEMENT_3D ( 'NONE', #6600, #935, #12160 ) ;
#10950=DIRECTION ( 'NONE',  ( -1.000000000000000000, 0.000000000000000000, 0.000000000000000000 ) ) ;
#10955=CARTESIAN_POINT ( 'NONE',  ( 10.19254911989241386, 23.71650635094626836, 80.00000000000000000 ) ) ;
#10960=ORIENTED_EDGE ( 'NONE', *, *, #7521, .T. ) ;
#10962=CARTESIAN_POINT ( 'NONE',  ( -0.9407811293054709756, 43.00000000000008527, 80.00000000000000000 ) ) ;
#10967=VECTOR ( 'NONE', #10239, 1000.000000000000114 ) ;
#10979=DIRECTION ( 'NONE',  ( 1.000000000000000000, 0.000000000000000000, 0.000000000000000000 ) ) ;
#10987=ORIENTED_EDGE ( 'NONE', *, *, #11628, .T. ) ;
#10990=ORIENTED_EDGE ( 'NONE', *, *, #214, .T. ) ;
#10993=EDGE_CURVE ( 'NONE', #6913, #9588, #5360, .T. ) ;
#10997=PLANE ( 'NONE',  #4113 ) ;
#11004=LINE ( 'NONE', #12077, #11431 ) ;
#11006=DIRECTION ( 'NONE',  ( 1.000000000000000000, 0.000000000000000000, 0.000000000000000000 ) ) ;
#11013=AXIS2_PLACEMENT_3D ( 'NONE', #4656, #12274, #7527 ) ;
#11015=DIRECTION ( 'NONE',  ( 1.224646799147353207E-16, 1.000000000000000000, -0.000000000000000000 ) ) ;
#11032=VECTOR ( 'NONE', #6293, 1000.000000000000000 ) ;
#11034=CARTESIAN_POINT ( 'NONE',  ( -1.440781129305282571, 17.00000000000009592, 79.50000000000000000 ) ) ;
#11046=ORIENTED_EDGE ( 'NONE', *, *, #12117, .F. ) ;
#11051=AXIS2_PLACEMENT_3D ( 'NONE', #8778, #2995, #6799 ) ;
#11055=EDGE_CURVE ( 'NONE', #4148, #938, #1786, .T. ) ;
#11064=VECTOR ( 'NONE', #6814, 1000.000000000000000 ) ;
#11067=EDGE_LOOP ( 'NONE', ( #8026, #6719, #9987, #11652 ) ) ;
#11071=AXIS2_PLACEMENT_3D ( 'NONE', #6874, #5700, #7859 ) ;
#11072=CARTESIAN_POINT ( 'NONE',  ( 9.942549119892413856, 23.28349364905404428, 79.50000000000000000 ) ) ;
#11074=LINE ( 'NONE', #2769, #4624 ) ;
#11077=CARTESIAN_POINT ( 'NONE',  ( 9.942549119892305498, 36.71650635094628967, 79.50000000000000000 ) ) ;
#11084=VECTOR ( 'NONE', #11824, 1000.000000000000114 ) ;
#11085=EDGE_CURVE ( 'NONE', #1902, #7629, #680, .T. ) ;
#11089=VERTEX_POINT ( 'NONE', #871 ) ;
#11093=CARTESIAN_POINT ( 'NONE',  ( -1.440781129305471087, 43.00000000000008527, 80.00000000000000000 ) ) ;
#11095=FACE_OUTER_BOUND ( 'NONE', #716, .T. ) ;
#11096=VERTEX_POINT ( 'NONE', #1796 ) ;
#11115=VECTOR ( 'NONE', #3733, 1000.000000000000114 ) ;
#11116=FACE_OUTER_BOUND ( 'NONE', #984, .T. ) ;
#11117=COLOUR_RGB ( '', 0.09019608, 0.27058824, 0.51372549) ;
#11119=ORIENTED_EDGE ( 'NONE', *, *, #1972, .F. ) ;
#11127=EDGE_CURVE ( 'NONE', #2311, #5671, #8209, .T. ) ;
#11128=EDGE_CURVE ( 'NONE', #11256, #2522, #6419, .T. ) ;
#11131=LINE ( 'NONE', #7395, #7535 ) ;
#11132=CARTESIAN_POINT ( 'NONE',  ( 9.984215786548631399, 23.35566243268464603, 80.00000048127353125 ) ) ;
#11133=EDGE_CURVE ( 'NONE', #632, #11972, #10205, .T. ) ;
#11134=CARTESIAN_POINT ( 'NONE',  ( -9.726035167149685634, 24.78349364905394125, 80.00000000000000000 ) ) ;
#11135=CARTESIAN_POINT ( 'NONE',  ( 7.344472908539098732, 24.78349364905406205, 80.00000000000000000 ) ) ;
#11137=LINE ( 'NONE', #5285, #8785 ) ;
#11146=ADVANCED_FACE ( 'NONE', ( #7476 ), #810, .T. ) ;
#11150=EDGE_LOOP ( 'NONE', ( #3484, #6302, #4425, #1262 ) ) ;
#11163=ORIENTED_EDGE ( 'NONE', *, *, #7214, .T. ) ;
#11169=AXIS2_PLACEMENT_3D ( 'NONE', #1403, #8991, #7196 ) ;
#11178=EDGE_LOOP ( 'NONE', ( #10935, #1361, #4351, #3302 ) ) ;
#11179=CARTESIAN_POINT ( 'NONE',  ( 11.80921887069467324, 29.75000000000018474, 80.00000000000000000 ) ) ;
#11184=ORIENTED_EDGE ( 'NONE', *, *, #4793, .F. ) ;
#11186=DIRECTION ( 'NONE',  ( 0.8660254037844365982, -0.5000000000000036637, 0.000000000000000000 ) ) ;
#11187=CARTESIAN_POINT ( 'NONE',  ( 11.80921887069467324, 29.75000000000018474, 79.50000000000000000 ) ) ;
#11189=ADVANCED_FACE ( 'NONE', ( #11095 ), #7417, .F. ) ;
#11195=LINE ( 'NONE', #10118, #5460 ) ;
#11199=CARTESIAN_POINT ( 'NONE',  ( 11.80921887069467324, 29.75000000000018474, 80.00000000000000000 ) ) ;
#11202=LINE ( 'NONE', #2535, #4912 ) ;
#11216=ORIENTED_EDGE ( 'NONE', *, *, #608, .F. ) ;
#11222=VECTOR ( 'NONE', #10514, 1000.000000000000000 ) ;
#11231=ORIENTED_EDGE ( 'NONE', *, *, #1926, .T. ) ;
#11236=CIRCLE ( 'NONE', #3857, 12.99999999999999822 ) ;
#11237=VECTOR ( 'NONE', #7545, 999.9999999999998863 ) ;
#11242=EDGE_CURVE ( 'NONE', #5677, #9755, #10641, .T. ) ;
#11243=B_SPLINE_CURVE_WITH_KNOTS ( 'NONE', 3,
 ( #12203, #7459, #4332, #1540 ),
 .UNSPECIFIED., .F., .F.,
 ( 4, 4 ),
 ( 0.0009573067811866343675, 0.001207306781186544276 ),
 .UNSPECIFIED. ) ;
#11244=ORIENTED_EDGE ( 'NONE', *, *, #10225, .F. ) ;
#11251=ORIENTED_EDGE ( 'NONE', *, *, #5344, .T. ) ;
#11253=CARTESIAN_POINT ( 'NONE',  ( -6.407287480251391720, 21.46474596215567487, 79.50000000000000000 ) ) ;
#11256=VERTEX_POINT ( 'NONE', #2046 ) ;
#11263=LINE ( 'NONE', #4580, #8028 ) ;
#11264=EDGE_CURVE ( 'NONE', #3440, #8327, #7939, .T. ) ;
#11266=CARTESIAN_POINT ( 'NONE',  ( -14.19078112930532853, 30.25000000000008882, 79.50000000000000000 ) ) ;
#11278=DIRECTION ( 'NONE',  ( 0.5000000000000036637, 0.8660254037844364872, 0.000000000000000000 ) ) ;
#11284=ORIENTED_EDGE ( 'NONE', *, *, #2567, .T. ) ;
#11297=AXIS2_PLACEMENT_3D ( 'NONE', #5330, #11186, #5578 ) ;
#11305=VERTEX_POINT ( 'NONE', #9575 ) ;
#11312=EDGE_CURVE ( 'NONE', #8405, #7265, #5972, .T. ) ;
#11323=VERTEX_POINT ( 'NONE', #6909 ) ;
#11324=DIRECTION ( 'NONE',  ( 7.011174048739587977E-15, 1.000000000000000000, 0.000000000000000000 ) ) ;
#11331=FACE_OUTER_BOUND ( 'NONE', #574, .T. ) ;
#11334=EDGE_CURVE ( 'NONE', #5535, #3208, #2174, .T. ) ;
#11335=CARTESIAN_POINT ( 'NONE',  ( -11.19078112930532498, 30.25000000000005684, 79.50000000000000000 ) ) ;
#11340=CARTESIAN_POINT ( 'NONE',  ( 9.942549119892413856, 23.28349364905404428, 79.50000000000000000 ) ) ;
#11344=ORIENTED_EDGE ( 'NONE', *, *, #214, .F. ) ;
#11346=VERTEX_POINT ( 'NONE', #6466 ) ;
#11351=DIRECTION ( 'NONE',  ( 0.000000000000000000, 0.000000000000000000, 1.000000000000000000 ) ) ;
#11352=VECTOR ( 'NONE', #5012, 1000.000000000000114 ) ;
#11364=EDGE_LOOP ( 'NONE', ( #6113, #3168, #8063, #1060, #9057 ) ) ;
#11366=CARTESIAN_POINT ( 'NONE',  ( -1.190781129305471087, 30.00000000000008882, 80.00000000000000000 ) ) ;
#11371=VERTEX_POINT ( 'NONE', #11562 ) ;
#11372=DIRECTION ( 'NONE',  ( -1.040834085586083310E-14, -1.000000000000000000, 0.000000000000000000 ) ) ;
#11376=ORIENTED_EDGE ( 'NONE', *, *, #5654, .T. ) ;
#11378=ADVANCED_FACE ( 'NONE', ( #4075 ), #3016, .T. ) ;
#11384=ORIENTED_EDGE ( 'NONE', *, *, #2427, .T. ) ;
#11385=AXIS2_PLACEMENT_3D ( 'NONE', #3375, #10151, #7173 ) ;
#11387=LINE ( 'NONE', #8437, #9356 ) ;
#11392=VECTOR ( 'NONE', #2717, 1000.000000000000000 ) ;
#11394=UNCERTAINTY_MEASURE_WITH_UNIT (LENGTH_MEASURE( 1.000000000000000082E-05 ), #967, 'distance_accuracy_value', 'NONE');
#11397=DIRECTION ( 'NONE',  ( -0.000000000000000000, -0.000000000000000000, 1.000000000000000000 ) ) ;
#11413=DIRECTION ( 'NONE',  ( 1.000000000000000000, 0.000000000000000000, 0.000000000000000000 ) ) ;
#11417=CARTESIAN_POINT ( 'NONE',  ( -1.190781129305471087, 30.00000000000008882, 78.00000000000000000 ) ) ;
#11423=VERTEX_POINT ( 'NONE', #8735 ) ;
#11431=VECTOR ( 'NONE', #7203, 1000.000000000000000 ) ;
#11436=PLANE ( 'NONE',  #10143 ) ;
#11440=EDGE_CURVE ( 'NONE', #11305, #3755, #12294, .T. ) ;
#11442=VECTOR ( 'NONE', #8239, 1000.000000000000227 ) ;
#11444=VECTOR ( 'NONE', #3300, 1000.000000000000114 ) ;
#11454=ORIENTED_EDGE ( 'NONE', *, *, #1655, .F. ) ;
#11458=FACE_OUTER_BOUND ( 'NONE', #11517, .T. ) ;
#11466=VECTOR ( 'NONE', #11278, 1000.000000000000114 ) ;
#11467=DIRECTION ( 'NONE',  ( 0.4999999999999878431, -0.8660254037844455910, 0.000000000000000000 ) ) ;
#11470=ORIENTED_EDGE ( 'NONE', *, *, #5883, .T. ) ;
#11473=VECTOR ( 'NONE', #1046, 1000.000000000000114 ) ;
#11475=CARTESIAN_POINT ( 'NONE',  ( 5.525725221640833240, 18.86666975080242992, 79.50000000000000000 ) ) ;
#11479=CARTESIAN_POINT ( 'NONE',  ( 9.940467135547230271, 36.71530431672421457, 80.00000000000000000 ) ) ;
#11480=FACE_OUTER_BOUND ( 'NONE', #10255, .T. ) ;
#11481=ORIENTED_EDGE ( 'NONE', *, *, #927, .F. ) ;
#11482=PRODUCT_CONTEXT ( 'NONE', #10425, 'mechanical' ) ;
#11484=AXIS2_PLACEMENT_3D ( 'NONE', #916, #5591, #855 ) ;
#11491=VERTEX_POINT ( 'NONE', #6006 ) ;
#11492=DIRECTION ( 'NONE',  ( -0.000000000000000000, 0.000000000000000000, 1.000000000000000000 ) ) ;
#11499=LINE ( 'NONE', #4887, #11064 ) ;
#11517=EDGE_LOOP ( 'NONE', ( #6589, #11344, #10338, #3337 ) ) ;
#11530=DIRECTION ( 'NONE',  ( 0.8660254037844331565, -0.5000000000000095479, 0.000000000000000000 ) ) ;
#11531=PRODUCT_DEFINITION_FORMATION_WITH_SPECIFIED_SOURCE ( 'ANY', '', #8455, .NOT_KNOWN. ) ;
#11536=LINE ( 'NONE', #297, #45 ) ;
#11541=EDGE_CURVE ( 'NONE', #11491, #3929, #12347, .T. ) ;
#11544=CARTESIAN_POINT ( 'NONE',  ( 8.809218870694669690, 29.75000000000019540, 79.50000000000000000 ) ) ;
#11549=VECTOR ( 'NONE', #5851, 1000.000000000000000 ) ;
#11551=CARTESIAN_POINT ( 'NONE',  ( 5.092712519748611832, 18.61666975080242992, 80.00000000000000000 ) ) ;
#11562=CARTESIAN_POINT ( 'NONE',  ( 5.092712519748452848, 41.38333024919784719, 80.00000000000000000 ) ) ;
#11570=ADVANCED_FACE ( 'NONE', ( #4369 ), #8230, .F. ) ;
#11576=VECTOR ( 'NONE', #6896, 1000.000000000000114 ) ;
#11580=ORIENTED_EDGE ( 'NONE', *, *, #3103, .T. ) ;
#11581=AXIS2_PLACEMENT_3D ( 'NONE', #8847, #1322, #5817 ) ;
#11586=DIRECTION ( 'NONE',  ( -0.000000000000000000, -1.000000000000000000, 0.000000000000000000 ) ) ;
#11587=VERTEX_POINT ( 'NONE', #3508 ) ;
#11599=ORIENTED_EDGE ( 'NONE', *, *, #11541, .T. ) ;
#11600=DIRECTION ( 'NONE',  ( 0.4999999999999985012, 0.8660254037844394848, 0.000000000000000000 ) ) ;
#11602=ORIENTED_EDGE ( 'NONE', *, *, #9744, .F. ) ;
#11608=CARTESIAN_POINT ( 'NONE',  ( 11.80921887069467324, 29.83333333331263049, 80.00000048127353125 ) ) ;
#11609=LINE ( 'NONE', #7732, #1621 ) ;
#11615=ORIENTED_EDGE ( 'NONE', *, *, #12206, .F. ) ;
#11624=FACE_OUTER_BOUND ( 'NONE', #11827, .T. ) ;
#11628=EDGE_CURVE ( 'NONE', #1631, #5677, #3321, .T. ) ;
#11630=ORIENTED_EDGE ( 'NONE', *, *, #8589, .F. ) ;
#11634=CARTESIAN_POINT ( 'NONE',  ( -1.190781129305471087, 30.00000000000008882, 80.00000000000000000 ) ) ;
#11636=CARTESIAN_POINT ( 'NONE',  ( -12.32411137850302119, 23.28349364905396612, 79.50000000000000000 ) ) ;
#11637=DIRECTION ( 'NONE',  ( 1.000000000000000000, 0.000000000000000000, 0.000000000000000000 ) ) ;
#11644=CARTESIAN_POINT ( 'NONE',  ( -7.907287480251421030, 41.13333024919781167, 79.50000000000000000 ) ) ;
#11648=DIRECTION ( 'NONE',  ( 1.000000000000000000, 0.000000000000000000, 0.000000000000000000 ) ) ;
#11652=ORIENTED_EDGE ( 'NONE', *, *, #7271, .F. ) ;
#11655=ADVANCED_FACE ( 'NONE', ( #4418 ), #3490, .T. ) ;
#11659=CARTESIAN_POINT ( 'NONE',  ( -12.32202939415815912, 36.71530431672423589, 80.00000000000000000 ) ) ;
#11661=ORIENTED_EDGE ( 'NONE', *, *, #2689, .F. ) ;
#11664=ORIENTED_EDGE ( 'NONE', *, *, #11264, .F. ) ;
#11672=ADVANCED_BREP_SHAPE_REPRESENTATION ( '', ( #8720, #1612 ), #4147 ) ;
#11678=LINE ( 'NONE', #3190, #6394 ) ;
#11679=CARTESIAN_POINT ( 'NONE',  ( -7.907287480251421030, 41.13333024919781167, 79.50000000000000000 ) ) ;
#11689=ORIENTED_EDGE ( 'NONE', *, *, #6942, .F. ) ;
#11697=AXIS2_PLACEMENT_3D ( 'NONE', #3824, #11372, #9606 ) ;
#11705=CARTESIAN_POINT ( 'NONE',  ( 0.000000000000000000, 0.000000000000000000, 79.50000000000000000 ) ) ;
#11712=CARTESIAN_POINT ( 'NONE',  ( 7.594472908538985045, 34.78349364905407270, 80.00000000000000000 ) ) ;
#11716=ORIENTED_EDGE ( 'NONE', *, *, #10287, .F. ) ;
#11719=ORIENTED_EDGE ( 'NONE', *, *, #713, .T. ) ;
#11721=CARTESIAN_POINT ( 'NONE',  ( 7.344472908539098732, 24.78349364905406205, 79.50000000000000000 ) ) ;
#11725=ORIENTED_EDGE ( 'NONE', *, *, #3275, .F. ) ;
#11727=ORIENTED_EDGE ( 'NONE', *, *, #7837, .T. ) ;
#11732=ORIENTED_EDGE ( 'NONE', *, *, #215, .T. ) ;
#11735=ORIENTED_EDGE ( 'NONE', *, *, #6920, .T. ) ;
#11742=AXIS2_PLACEMENT_3D ( 'NONE', #2551, #6597, #10393 ) ;
#11758=CARTESIAN_POINT ( 'NONE',  ( -14.19078112930533209, 29.75000000000008882, 79.50000000000000000 ) ) ;
#11759=LINE ( 'NONE', #399, #531 ) ;
#11763=EDGE_CURVE ( 'NONE', #1199, #6472, #8152, .T. ) ;
#11773=VECTOR ( 'NONE', #1205, 1000.000000000000000 ) ;
#11779=ORIENTED_EDGE ( 'NONE', *, *, #9142, .T. ) ;
#11781=EDGE_CURVE ( 'NONE', #10546, #9044, #4725, .T. ) ;
#11797=EDGE_CURVE ( 'NONE', #4222, #8405, #3611, .T. ) ;
#11816=ORIENTED_EDGE ( 'NONE', *, *, #11440, .F. ) ;
#11818=CARTESIAN_POINT ( 'NONE',  ( 11.80921887069467324, 30.25000000000018474, 80.00000000000000000 ) ) ;
#11822=LINE ( 'NONE', #8927, #5236 ) ;
#11824=DIRECTION ( 'NONE',  ( 0.8660254037844331565, -0.5000000000000095479, 0.000000000000000000 ) ) ;
#11827=EDGE_LOOP ( 'NONE', ( #5608, #9950, #4946, #5418 ) ) ;
#11829=CARTESIAN_POINT ( 'NONE',  ( 10.06754911989233392, 36.50000000000012079, 80.00000000000000000 ) ) ;
#11844=VERTEX_POINT ( 'NONE', #8518 ) ;
#11846=VERTEX_POINT ( 'NONE', #12342 ) ;
#11853=ADVANCED_FACE ( 'NONE', ( #1680 ), #9453, .T. ) ;
#11854=VECTOR ( 'NONE', #10527, 1000.000000000000000 ) ;
#11857=CIRCLE ( 'NONE', #6664, 14.99999999999999822 ) ;
#11861=ORIENTED_EDGE ( 'NONE', *, *, #10287, .T. ) ;
#11864=DIRECTION ( 'NONE',  ( -0.000000000000000000, -1.000000000000000000, 0.000000000000000000 ) ) ;
#11866=PLANE ( 'NONE',  #8029 ) ;
#11873=AXIS2_PLACEMENT_3D ( 'NONE', #10517, #9757, #6718 ) ;
#11891=CARTESIAN_POINT ( 'NONE',  ( -14.19078112930533031, 30.00000000000017764, 80.00000000000000000 ) ) ;
#11899=DIRECTION ( 'NONE',  ( 1.000000000000000000, -1.040834085586083310E-14, 0.000000000000000000 ) ) ;
#11908=CARTESIAN_POINT ( 'NONE',  ( 5.381387654344468530, 41.21666358253047946, 80.00000000000000000 ) ) ;
#11909=ORIENTED_EDGE ( 'NONE', *, *, #3072, .F. ) ;
#11916=EDGE_CURVE ( 'NONE', #2084, #6749, #7355, .T. ) ;
#11920=CARTESIAN_POINT ( 'NONE',  ( -1.190781129305471087, 30.00000000000008882, 65.00000000000000000 ) ) ;
#11921=ORIENTED_EDGE ( 'NONE', *, *, #10770, .F. ) ;
#11924=VECTOR ( 'NONE', #467, 1000.000000000000114 ) ;
#11925=EDGE_LOOP ( 'NONE', ( #624, #636, #2250, #8401, #1923, #8679, #2145, #5268, #10351, #12056, #7724, #12133, #2000, #11376, #3377, #4133, #5381, #7598, #1984, #1931, #2216, #6367, #7471, #5724, #8111, #2435, #2126, #3512, #11719, #7915, #11978, #10922, #11664 ) ) ;
#11927=LINE ( 'NONE', #4072, #3525 ) ;
#11928=DIRECTION ( 'NONE',  ( -0.5000000000000006661, -0.8660254037844383745, 0.000000000000000000 ) ) ;
#11935=PLANE ( 'NONE',  #496 ) ;
#11948=EDGE_CURVE ( 'NONE', #3208, #5427, #1118, .T. ) ;
#11958=ORIENTED_EDGE ( 'NONE', *, *, #8645, .T. ) ;
#11964=LINE ( 'NONE', #10955, #7225 ) ;
#11969=VERTEX_POINT ( 'NONE', #7836 ) ;
#11972=VERTEX_POINT ( 'NONE', #3856 ) ;
#11978=ORIENTED_EDGE ( 'NONE', *, *, #643, .F. ) ;
#11979=ORIENTED_EDGE ( 'NONE', *, *, #968, .T. ) ;
#11988=VERTEX_POINT ( 'NONE', #169 ) ;
#11998=ORIENTED_EDGE ( 'NONE', *, *, #4088, .T. ) ;
#12006=ORIENTED_EDGE ( 'NONE', *, *, #6789, .T. ) ;
#12010=PLANE ( 'NONE',  #8828 ) ;
#12014=CARTESIAN_POINT ( 'NONE',  ( -12.32411137850302119, 23.28349364905396612, 79.50000000000000000 ) ) ;
#12025=DIRECTION ( 'NONE',  ( -0.000000000000000000, -0.000000000000000000, 1.000000000000000000 ) ) ;
#12027=VECTOR ( 'NONE', #3766, 1000.000000000000227 ) ;
#12031=PLANE ( 'NONE',  #4874 ) ;
#12033=EDGE_CURVE ( 'NONE', #7550, #1521, #1237, .T. ) ;
#12040=CARTESIAN_POINT ( 'NONE',  ( -7.690781129305457320, 18.74166975080245834, 80.00000000000000000 ) ) ;
#12042=VERTEX_POINT ( 'NONE', #11712 ) ;
#12044=FACE_OUTER_BOUND ( 'NONE', #6923, .T. ) ;
#12052=CARTESIAN_POINT ( 'NONE',  ( -1.190781129305471087, 30.00000000000008882, 80.00000000000000000 ) ) ;
#12056=ORIENTED_EDGE ( 'NONE', *, *, #11334, .F. ) ;
#12059=ORIENTED_EDGE ( 'NONE', *, *, #10184, .F. ) ;
#12065=CARTESIAN_POINT ( 'NONE',  ( 3.592712519748626931, 21.21474596215575659, 79.50000000000000000 ) ) ;
#12077=CARTESIAN_POINT ( 'NONE',  ( 11.80921887069467324, 30.25000000000018474, 80.00000000000000000 ) ) ;
#12079=CARTESIAN_POINT ( 'NONE',  ( 10.06754911989234635, 23.50000000000004974, 80.00000000000000000 ) ) ;
#12082=DIRECTION ( 'NONE',  ( 0.8660254037844434816, 0.4999999999999913958, 0.000000000000000000 ) ) ;
#12099=ORIENTED_EDGE ( 'NONE', *, *, #12033, .T. ) ;
#12108=LINE ( 'NONE', #10634, #6407 ) ;
#12110=ORIENTED_EDGE ( 'NONE', *, *, #7393, .F. ) ;
#12115=DIRECTION ( 'NONE',  ( -0.8660254037844377084, 0.5000000000000015543, 0.000000000000000000 ) ) ;
#12117=EDGE_CURVE ( 'NONE', #2446, #3205, #8761, .T. ) ;
#12118=ADVANCED_FACE ( 'NONE', ( #8015 ), #8137, .T. ) ;
#12119=VERTEX_POINT ( 'NONE', #2480 ) ;
#12120=VECTOR ( 'NONE', #9641, 1000.000000000000114 ) ;
#12133=ORIENTED_EDGE ( 'NONE', *, *, #5948, .T. ) ;
#12135=EDGE_CURVE ( 'NONE', #7067, #11423, #10827, .T. ) ;
#12142=CARTESIAN_POINT ( 'NONE',  ( -0.9407811293054709756, 40.00000000000008527, 79.50000000000000000 ) ) ;
#12143=CARTESIAN_POINT ( 'NONE',  ( -7.474274778359198734, 41.38333024919781167, 79.50000000000000000 ) ) ;
#12156=CARTESIAN_POINT ( 'NONE',  ( -12.32202939415814846, 23.28469568327592754, 80.00000000000000000 ) ) ;
#12160=DIRECTION ( 'NONE',  ( 1.000000000000000000, 0.000000000000000000, 0.000000000000000000 ) ) ;
#12175=DIRECTION ( 'NONE',  ( -0.5000000000000036637, -0.8660254037844365982, 0.000000000000000000 ) ) ;
#12187=LINE ( 'NONE', #8541, #5469 ) ;
#12188=CARTESIAN_POINT ( 'NONE',  ( -1.190781129305471087, 30.00000000000008882, 80.00000000000000000 ) ) ;
#12191=DIRECTION ( 'NONE',  ( -0.8660254037844394848, -0.4999999999999985012, 0.000000000000000000 ) ) ;
#12192=AXIS2_PLACEMENT_3D ( 'NONE', #1170, #9692, #4972 ) ;
#12197=VERTEX_POINT ( 'NONE', #1421 ) ;
#12198=EDGE_CURVE ( 'NONE', #5570, #10546, #542, .T. ) ;
#12203=CARTESIAN_POINT ( 'NONE',  ( -14.19078112930533031, 30.00000000000017764, 80.00000000000000000 ) ) ;
#12206=EDGE_CURVE ( 'NONE', #2842, #10602, #4467, .T. ) ;
#12214=CARTESIAN_POINT ( 'NONE',  ( -12.49077804517044221, 23.57216878365009194, 80.00000000000000000 ) ) ;
#12216=AXIS2_PLACEMENT_3D ( 'NONE', #1549, #4287, #5354 ) ;
#12220=DIRECTION ( 'NONE',  ( -0.4999999999999970579, 0.8660254037844403729, 0.000000000000000000 ) ) ;
#12236=VECTOR ( 'NONE', #9801, 1000.000000000000227 ) ;
#12244=SHAPE_REPRESENTATION ( 'Pulse _ Speed Control Dial', ( #1612 ), #4147 ) ;
#12259=ORIENTED_EDGE ( 'NONE', *, *, #2273, .T. ) ;
#12261=LINE ( 'NONE', #3708, #41 ) ;
#12262=VECTOR ( 'NONE', #5340, 1000.000000000000000 ) ;
#12266=ORIENTED_EDGE ( 'NONE', *, *, #11797, .T. ) ;
#12274=DIRECTION ( 'NONE',  ( 1.000000000000000000, -0.000000000000000000, 0.000000000000000000 ) ) ;
#12286=LINE ( 'NONE', #8583, #11115 ) ;
#12294=B_SPLINE_CURVE_WITH_KNOTS ( 'NONE', 3,
 ( #3198, #7867, #2080, #264 ),
 .UNSPECIFIED., .F., .F.,
 ( 4, 4 ),
 ( 0.0002502309401075617249, 0.0005002309401076790408 ),
 .UNSPECIFIED. ) ;
#12296=DIRECTION ( 'NONE',  ( 0.000000000000000000, -0.000000000000000000, -1.000000000000000000 ) ) ;
#12302=LINE ( 'NONE', #2132, #3771 ) ;
#12309=DIRECTION ( 'NONE',  ( -0.5000000000000016653, -0.8660254037844378194, 0.000000000000000000 ) ) ;
#12311=DIRECTION ( 'NONE',  ( -0.000000000000000000, -0.000000000000000000, 1.000000000000000000 ) ) ;
#12324=PLANE ( 'NONE',  #11051 ) ;
#12326=ADVANCED_FACE ( 'NONE', ( #11331 ), #739, .T. ) ;
#12337=DIRECTION ( 'NONE',  ( 0.4999999999999914513, -0.8660254037844435926, 0.000000000000000000 ) ) ;
#12341=VERTEX_POINT ( 'NONE', #2541 ) ;
#12342=CARTESIAN_POINT ( 'NONE',  ( 5.525725221640833240, 18.86666975080242992, 80.00000000000000000 ) ) ;
#12343=EDGE_CURVE ( 'NONE', #12042, #7445, #10129, .T. ) ;
#12346=DIRECTION ( 'NONE',  ( -0.8660254037844394848, -0.4999999999999985012, 0.000000000000000000 ) ) ;
#12347=CIRCLE ( 'NONE', #8753, 12.99999999999999822 ) ;
ENDSEC;
END-ISO-10303-21;
